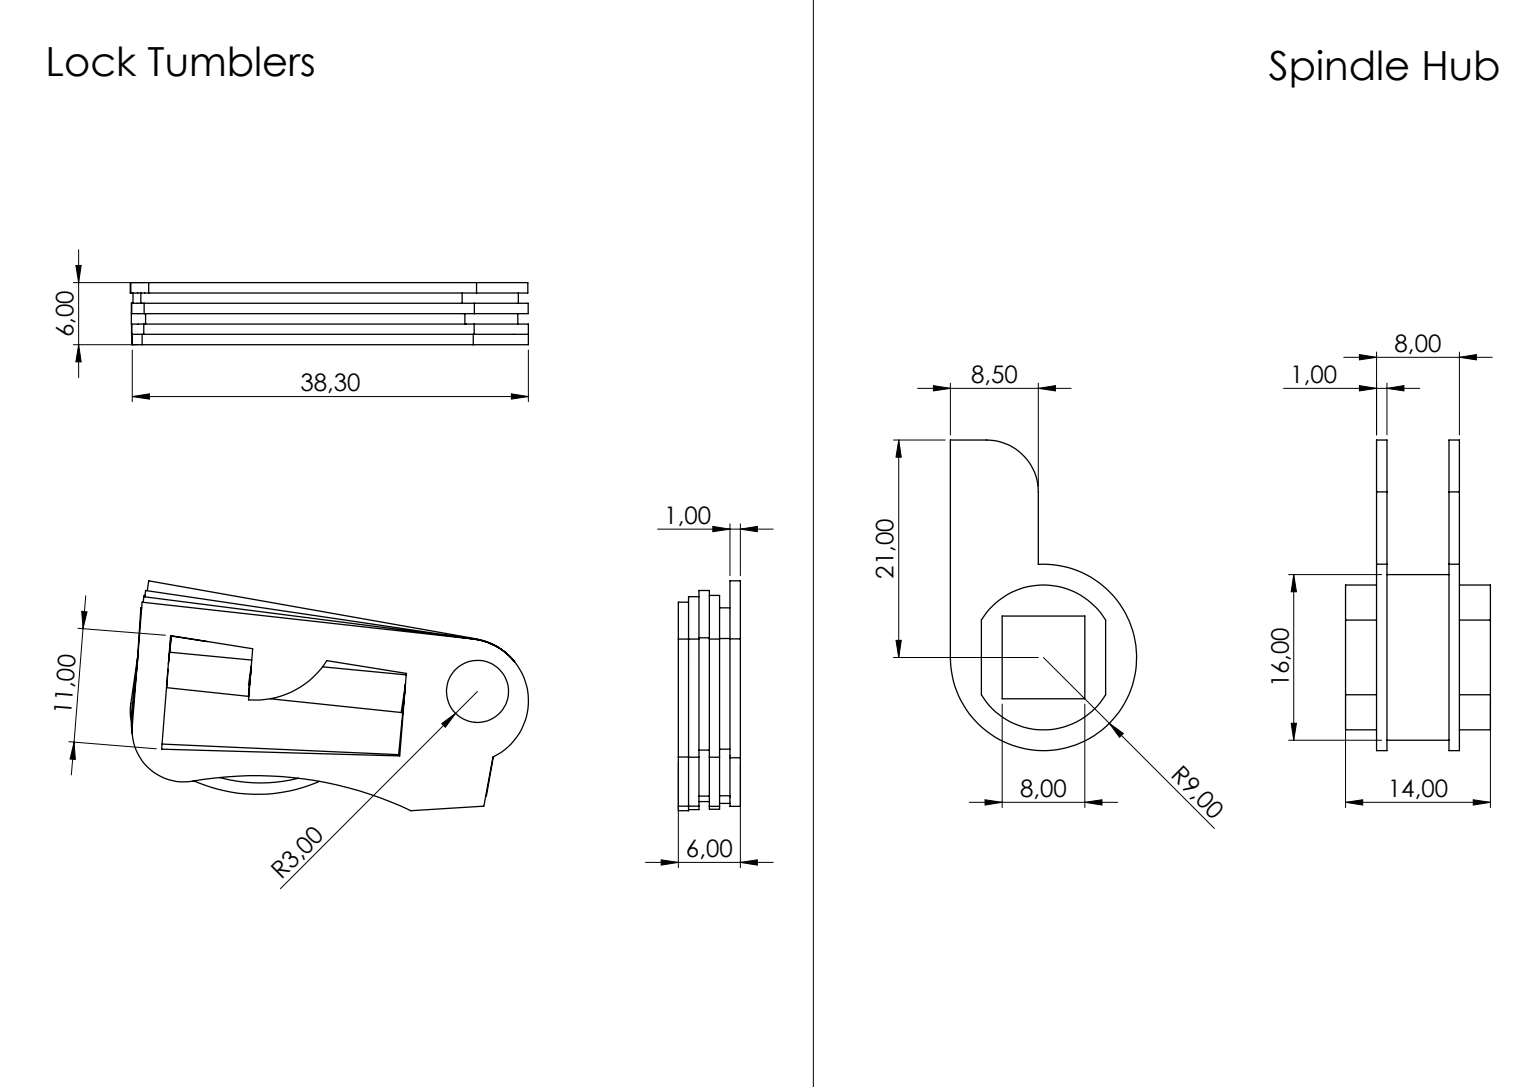
ISO-10303-21;
HEADER;
FILE_DESCRIPTION (('STEP AP214'),
    '1' );
FILE_NAME ('Lock Tumblers.step',
    '2026-10-06T13:23:30',
    ( '' ),
    ( '' ),
    'SwSTEP 2.0',
    'SolidWorks 2020',
    '' );
FILE_SCHEMA (( 'AUTOMOTIVE_DESIGN' ));
ENDSEC;

DATA;
#9=LINE ( 'NONE', #19761, #1381 ) ;
#17=VECTOR ( 'NONE', #19861, 1000.000000000000114 ) ;
#19=EDGE_CURVE ( 'NONE', #10851, #14365, #21344, .T. ) ;
#28=LINE ( 'NONE', #12848, #13253 ) ;
#29=DIRECTION ( 'NONE',  ( -2.842170943040000002E-14, -3.552713678800000097E-13, -1.000000000000000000 ) ) ;
#30=VERTEX_POINT ( 'NONE', #23278 ) ;
#34=VERTEX_POINT ( 'NONE', #8858 ) ;
#37=CARTESIAN_POINT ( 'NONE',  ( 5.631397321050000571, -17.85059010000000157, -146.5552959529999839 ) ) ;
#50=EDGE_CURVE ( 'NONE', #22537, #320, #23237, .T. ) ;
#60=AXIS2_PLACEMENT_3D ( 'NONE', #23173, #12444, #1408 ) ;
#64=LINE ( 'NONE', #5521, #16191 ) ;
#66=PLANE ( 'NONE',  #21173 ) ;
#67=CARTESIAN_POINT ( 'NONE',  ( 15.97954986339999905, -26.72957102550000030, -142.5552959529999839 ) ) ;
#69=CARTESIAN_POINT ( 'NONE',  ( -4.946601369560000627, -23.77962690289999870, -143.5552959529999839 ) ) ;
#80=CARTESIAN_POINT ( 'NONE',  ( 1.600095057559999923, -18.40127899619999852, -146.5552959529999839 ) ) ;
#81=VECTOR ( 'NONE', #14435, 1000.000000000000114 ) ;
#82=ORIENTED_EDGE ( 'NONE', *, *, #12596, .T. ) ;
#87=ORIENTED_EDGE ( 'NONE', *, *, #14036, .T. ) ;
#93=DIRECTION ( 'NONE',  ( -0.9892101392001054760, 0.1465035852930155480, 4.471739159800472250E-12 ) ) ;
#97=AXIS2_PLACEMENT_3D ( 'NONE', #8071, #2741, #23074 ) ;
#98=EDGE_CURVE ( 'NONE', #6545, #18690, #5646, .T. ) ;
#101=ORIENTED_EDGE ( 'NONE', *, *, #18336, .T. ) ;
#109=EDGE_CURVE ( 'NONE', #2866, #16847, #2210, .T. ) ;
#115=FACE_OUTER_BOUND ( 'NONE', #19032, .T. ) ;
#117=CARTESIAN_POINT ( 'NONE',  ( -4.959431410700000598, -23.66636161550000139, -146.0552959529999839 ) ) ;
#118=AXIS2_PLACEMENT_3D ( 'NONE', #14379, #10436, #6880 ) ;
#121=ORIENTED_EDGE ( 'NONE', *, *, #3001, .T. ) ;
#122=CARTESIAN_POINT ( 'NONE',  ( -4.160432423080000497, -28.71743394529999804, -144.5552959529999839 ) ) ;
#124=ORIENTED_EDGE ( 'NONE', *, *, #13380, .T. ) ;
#125=LINE ( 'NONE', #11042, #20030 ) ;
#129=DIRECTION ( 'NONE',  ( -0.9896415801065050477, 0.1435602414469278887, 8.992806499463764746E-12 ) ) ;
#133=CARTESIAN_POINT ( 'NONE',  ( 5.631397321050000571, -17.85059010000000157, -146.5552959529999839 ) ) ;
#152=PLANE ( 'NONE',  #286 ) ;
#164=CARTESIAN_POINT ( 'NONE',  ( -9.056357402059999728, -12.43025388040000045, -147.5552959529999839 ) ) ;
#173=DIRECTION ( 'NONE',  ( -0.09606172499277214338, -0.9953753789357123738, 8.234154099303244678E-13 ) ) ;
#177=EDGE_CURVE ( 'NONE', #22553, #21627, #7661, .T. ) ;
#189=ORIENTED_EDGE ( 'NONE', *, *, #7703, .T. ) ;
#207=ORIENTED_EDGE ( 'NONE', *, *, #948, .T. ) ;
#215=ORIENTED_EDGE ( 'NONE', *, *, #20592, .F. ) ;
#218=LINE ( 'NONE', #15834, #14813 ) ;
#222=ADVANCED_FACE ( 'NONE', ( #11458 ), #4098, .F. ) ;
#224=ORIENTED_EDGE ( 'NONE', *, *, #1037, .F. ) ;
#233=CARTESIAN_POINT ( 'NONE',  ( -6.601136089949999786, -20.10368962670000315, -144.5552959529999839 ) ) ;
#243=CARTESIAN_POINT ( 'NONE',  ( -9.347107914279998653, -17.32706600430000066, -144.5552959529999839 ) ) ;
#245=VECTOR ( 'NONE', #2038, 1000.000000000000114 ) ;
#249=LINE ( 'NONE', #5710, #16739 ) ;
#257=LINE ( 'NONE', #7499, #9038 ) ;
#259=VECTOR ( 'NONE', #18453, 1000.000000000000114 ) ;
#263=CARTESIAN_POINT ( 'NONE',  ( -9.923478264230000789, -23.29931827799999766, -144.5552959529999839 ) ) ;
#265=PLANE ( 'NONE',  #18891 ) ;
#272=VECTOR ( 'NONE', #12599, 1000.000000000000227 ) ;
#275=FACE_OUTER_BOUND ( 'NONE', #1405, .T. ) ;
#286=AXIS2_PLACEMENT_3D ( 'NONE', #3950, #12631, #10950 ) ;
#287=CARTESIAN_POINT ( 'NONE',  ( -9.969904307360000217, -22.67446893780000039, -144.5552959529999839 ) ) ;
#302=EDGE_LOOP ( 'NONE', ( #10238, #8735, #12930, #17915, #645, #16858 ) ) ;
#303=EDGE_CURVE ( 'NONE', #11439, #22823, #3876, .T. ) ;
#320=VERTEX_POINT ( 'NONE', #3034 ) ;
#323=FACE_OUTER_BOUND ( 'NONE', #460, .T. ) ;
#324=ORIENTED_EDGE ( 'NONE', *, *, #8627, .T. ) ;
#325=CARTESIAN_POINT ( 'NONE',  ( -9.434278515689999978, -18.41834002140000237, -147.5552959529999839 ) ) ;
#332=ADVANCED_FACE ( 'NONE', ( #22541 ), #3148, .T. ) ;
#342=DIRECTION ( 'NONE',  ( 0.02818224575639410520, 0.9996028016287901163, -8.199401781418279957E-13 ) ) ;
#343=VECTOR ( 'NONE', #12000, 1000.000000000000000 ) ;
#345=ORIENTED_EDGE ( 'NONE', *, *, #18029, .T. ) ;
#353=AXIS2_PLACEMENT_3D ( 'NONE', #12297, #17774, #23258 ) ;
#356=CARTESIAN_POINT ( 'NONE',  ( -8.296392858609999976, -9.821782169089999570, -148.5552959529999839 ) ) ;
#361=VERTEX_POINT ( 'NONE', #4450 ) ;
#369=DIRECTION ( 'NONE',  ( -2.839308199620000013E-14, -3.568879590630000244E-13, -1.000000000000000000 ) ) ;
#370=ORIENTED_EDGE ( 'NONE', *, *, #23215, .F. ) ;
#377=EDGE_CURVE ( 'NONE', #16716, #11246, #12757, .T. ) ;
#400=CIRCLE ( 'NONE', #3432, 2.999999999999999112 ) ;
#401=ORIENTED_EDGE ( 'NONE', *, *, #15313, .F. ) ;
#404=VERTEX_POINT ( 'NONE', #21825 ) ;
#405=CYLINDRICAL_SURFACE ( 'NONE', #14494, 8.176568160360000448 ) ;
#410=CARTESIAN_POINT ( 'NONE',  ( -7.129475577410000042, -25.57825421080000083, -144.0552959529999839 ) ) ;
#428=AXIS2_PLACEMENT_3D ( 'NONE', #17687, #19484, #10762 ) ;
#440=ADVANCED_FACE ( 'NONE', ( #21467 ), #14562, .T. ) ;
#449=ORIENTED_EDGE ( 'NONE', *, *, #3663, .T. ) ;
#451=ORIENTED_EDGE ( 'NONE', *, *, #12079, .F. ) ;
#456=LINE ( 'NONE', #20555, #2007 ) ;
#460=EDGE_LOOP ( 'NONE', ( #22587, #8189, #13653, #11072, #16704 ) ) ;
#463=VECTOR ( 'NONE', #13106, 999.9999999999998863 ) ;
#470=EDGE_CURVE ( 'NONE', #2284, #2388, #4261, .T. ) ;
#473=VERTEX_POINT ( 'NONE', #1610 ) ;
#475=ADVANCED_FACE ( 'NONE', ( #8830 ), #16110, .F. ) ;
#478=FACE_OUTER_BOUND ( 'NONE', #722, .T. ) ;
#490=LINE ( 'NONE', #2397, #14405 ) ;
#494=DIRECTION ( 'NONE',  ( 8.955190032050000935E-12, -9.104778821549999739E-13, 1.000000000000000000 ) ) ;
#496=ORIENTED_EDGE ( 'NONE', *, *, #9897, .T. ) ;
#497=EDGE_CURVE ( 'NONE', #7372, #10073, #14436, .T. ) ;
#498=MECHANICAL_DESIGN_GEOMETRIC_PRESENTATION_REPRESENTATION('',(#20638),#15318);
#512=ADVANCED_FACE ( 'NONE', ( #5969 ), #11083, .F. ) ;
#513=EDGE_CURVE ( 'NONE', #11545, #10772, #7749, .T. ) ;
#516=PRODUCT_DEFINITION_FORMATION_WITH_SPECIFIED_SOURCE ( 'ANY', '', #19655, .NOT_KNOWN. ) ;
#518=ORIENTED_EDGE ( 'NONE', *, *, #18360, .T. ) ;
#530=CARTESIAN_POINT ( 'NONE',  ( -6.547730170579999509, -18.66441632429999942, -147.5552959529999839 ) ) ;
#552=VECTOR ( 'NONE', #14058, 1000.000000000000000 ) ;
#558=DIRECTION ( 'NONE',  ( 0.05349466063429310358, 0.9985681355238719137, -1.093104632299860501E-13 ) ) ;
#561=ORIENTED_EDGE ( 'NONE', *, *, #19, .F. ) ;
#569=CARTESIAN_POINT ( 'NONE',  ( 4.352290413739999586, -26.01556969399999986, -145.5552959529999839 ) ) ;
#574=EDGE_CURVE ( 'NONE', #10851, #1178, #9171, .T. ) ;
#578=CARTESIAN_POINT ( 'NONE',  ( -6.264930628975839966, -16.71491984542973341, -147.5552959529461816 ) ) ;
#579=VECTOR ( 'NONE', #12352, 1000.000000000000114 ) ;
#580=DIRECTION ( 'NONE',  ( 1.000000000000000000, 0.000000000000000000, -1.522591576628786004E-13 ) ) ;
#588=ORIENTED_EDGE ( 'NONE', *, *, #13323, .F. ) ;
#589=LINE ( 'NONE', #22831, #9470 ) ;
#593=LINE ( 'NONE', #4279, #23134 ) ;
#599=DIRECTION ( 'NONE',  ( 4.430318231640945063E-12, -6.100259101492280662E-13, 1.000000000000000000 ) ) ;
#619=DIRECTION ( 'NONE',  ( -1.525446435830000185E-13, -8.171241461240000022E-13, -1.000000000000000000 ) ) ;
#621=DIRECTION ( 'NONE',  ( 1.000000000000000000, 0.000000000000000000, -4.510774274160000731E-12 ) ) ;
#622=FACE_OUTER_BOUND ( 'NONE', #19220, .T. ) ;
#627=DIRECTION ( 'NONE',  ( 0.9990052710704846461, -0.04459224566432164194, -1.160036675700561719E-13 ) ) ;
#632=VECTOR ( 'NONE', #2081, 1000.000000000000114 ) ;
#642=DIRECTION ( 'NONE',  ( 0.9990052710704846461, -0.04459224566432164194, -1.160036675700561719E-13 ) ) ;
#645=ORIENTED_EDGE ( 'NONE', *, *, #21775, .T. ) ;
#655=DIRECTION ( 'NONE',  ( 2.839308199620000013E-14, 3.568879590630000244E-13, 1.000000000000000000 ) ) ;
#667=ORIENTED_EDGE ( 'NONE', *, *, #18339, .F. ) ;
#672=LINE ( 'NONE', #8257, #20839 ) ;
#674=EDGE_LOOP ( 'NONE', ( #13508, #15033, #13775, #6801 ) ) ;
#685=ORIENTED_EDGE ( 'NONE', *, *, #13914, .T. ) ;
#689=LINE ( 'NONE', #22455, #8666 ) ;
#694=AXIS2_PLACEMENT_3D ( 'NONE', #20611, #4769, #621 ) ;
#698=ORIENTED_EDGE ( 'NONE', *, *, #6854, .T. ) ;
#701=CARTESIAN_POINT ( 'NONE',  ( -9.282104535849999394, -16.71402168319999859, -144.5552959529999839 ) ) ;
#703=DIRECTION ( 'NONE',  ( 0.1000233216789610108, 0.9949850929136109245, -3.588240815588595806E-13 ) ) ;
#712=VERTEX_POINT ( 'NONE', #6671 ) ;
#720=CARTESIAN_POINT ( 'NONE',  ( 24.89581725840000104, -26.85672394480000236, -144.5552959529999839 ) ) ;
#722=EDGE_LOOP ( 'NONE', ( #8412, #1698, #20815, #12753, #12822 ) ) ;
#727=ORIENTED_EDGE ( 'NONE', *, *, #8627, .F. ) ;
#732=DIRECTION ( 'NONE',  ( 1.527666881879999979E-13, 8.171241461240000022E-13, 1.000000000000000000 ) ) ;
#735=CARTESIAN_POINT ( 'NONE',  ( 25.00000852249999994, -26.83294714660000224, -143.5552959529999839 ) ) ;
#737=EDGE_CURVE ( 'NONE', #2750, #10162, #17272, .T. ) ;
#744=EDGE_CURVE ( 'NONE', #22823, #11439, #6921, .T. ) ;
#747=DIRECTION ( 'NONE',  ( 0.9944529286486341046, -0.1051825684329612265, -4.469111776238355154E-12 ) ) ;
#749=CARTESIAN_POINT ( 'NONE',  ( 23.40529971389999986, -31.60139774330000151, -148.5552959529999839 ) ) ;
#753=AXIS2_PLACEMENT_3D ( 'NONE', #701, #11861, #18779 ) ;
#757=CIRCLE ( 'NONE', #2659, 9.999999999999998224 ) ;
#760=VERTEX_POINT ( 'NONE', #3003 ) ;
#773=DIRECTION ( 'NONE',  ( 1.000000000000000000, 0.000000000000000000, -4.429789868254375404E-12 ) ) ;
#776=AXIS2_PLACEMENT_3D ( 'NONE', #3674, #5214, #14152 ) ;
#792=EDGE_CURVE ( 'NONE', #34, #13141, #18820, .T. ) ;
#799=ADVANCED_FACE ( 'NONE', ( #15723 ), #13459, .T. ) ;
#803=DIRECTION ( 'NONE',  ( 8.955190032048950803E-12, -9.104778821523669707E-13, 1.000000000000000000 ) ) ;
#807=VECTOR ( 'NONE', #9050, 1000.000000000000227 ) ;
#808=ORIENTED_EDGE ( 'NONE', *, *, #13766, .F. ) ;
#811=DIRECTION ( 'NONE',  ( 1.000000000000000000, 0.000000000000000000, -8.953948693601887499E-12 ) ) ;
#817=DIRECTION ( 'NONE',  ( -0.9968185442904001770, 0.07970438983373183406, 8.881784197001251061E-14 ) ) ;
#819=EDGE_CURVE ( 'NONE', #5226, #404, #5017, .T. ) ;
#821=ADVANCED_FACE ( 'NONE', ( #16081 ), #23100, .T. ) ;
#832=DIRECTION ( 'NONE',  ( -0.1739442350240419932, -0.9847555042252370550, 8.300754441162000146E-13 ) ) ;
#833=EDGE_LOOP ( 'NONE', ( #16768, #6878, #10888, #18161, #3058, #10823 ) ) ;
#834=PLANE ( 'NONE',  #6066 ) ;
#836=ORIENTED_EDGE ( 'NONE', *, *, #936, .F. ) ;
#842=CARTESIAN_POINT ( 'NONE',  ( -9.157754307299999397, -15.75963164970000108, -148.5552959529999839 ) ) ;
#846=DIRECTION ( 'NONE',  ( -0.07970438983373200059, -0.9968185442904001770, 8.268372250843320857E-13 ) ) ;
#852=DIRECTION ( 'NONE',  ( 1.526468026909860048E-13, 8.159623473498529972E-13, 1.000000000000000000 ) ) ;
#854=EDGE_CURVE ( 'NONE', #14669, #14970, #11031, .T. ) ;
#859=DIRECTION ( 'NONE',  ( 0.000000000000000000, -1.000000000000000000, 8.159623473500000156E-13 ) ) ;
#865=VECTOR ( 'NONE', #15700, 1000.000000000000000 ) ;
#866=DIRECTION ( 'NONE',  ( 0.000000000000000000, 1.093106450072369968E-12, -1.000000000000000000 ) ) ;
#874=ORIENTED_EDGE ( 'NONE', *, *, #177, .T. ) ;
#888=DIRECTION ( 'NONE',  ( -0.9892101392001054760, 0.1465035852930155480, 4.471739159800472250E-12 ) ) ;
#890=LINE ( 'NONE', #6109, #6665 ) ;
#900=ORIENTED_EDGE ( 'NONE', *, *, #13310, .T. ) ;
#914=CARTESIAN_POINT ( 'NONE',  ( 24.11847952820000174, -31.58456057200000089, -143.0552959529999839 ) ) ;
#917=ORIENTED_EDGE ( 'NONE', *, *, #16657, .T. ) ;
#919=VERTEX_POINT ( 'NONE', #10579 ) ;
#922=ORIENTED_EDGE ( 'NONE', *, *, #6201, .F. ) ;
#923=AXIS2_PLACEMENT_3D ( 'NONE', #3964, #20620, #5970 ) ;
#929=DIRECTION ( 'NONE',  ( 0.9957290851625899553, -0.09232328504376198508, -9.001390970786290700E-12 ) ) ;
#930=ORIENTED_EDGE ( 'NONE', *, *, #18567, .F. ) ;
#936=EDGE_CURVE ( 'NONE', #19018, #10871, #218, .T. ) ;
#948=EDGE_CURVE ( 'NONE', #8156, #9207, #7576, .T. ) ;
#955=CARTESIAN_POINT ( 'NONE',  ( 2.218297500559999857, -15.44723318490000175, -146.5552959529999839 ) ) ;
#956=EDGE_CURVE ( 'NONE', #22736, #2628, #6149, .T. ) ;
#959=EDGE_CURVE ( 'NONE', #19705, #16855, #22573, .T. ) ;
#960=CARTESIAN_POINT ( 'NONE',  ( 1.829659965300000080, -16.02499107890000118, -143.5552959529999839 ) ) ;
#961=AXIS2_PLACEMENT_3D ( 'NONE', #19818, #21604, #5064 ) ;
#962=ORIENTED_EDGE ( 'NONE', *, *, #13286, .T. ) ;
#966=LINE ( 'NONE', #6082, #22322 ) ;
#975=VECTOR ( 'NONE', #19311, 1000.000000000000114 ) ;
#976=ORIENTED_EDGE ( 'NONE', *, *, #17520, .F. ) ;
#987=DIRECTION ( 'NONE',  ( 0.000000000000000000, 1.093106450072369968E-12, -1.000000000000000000 ) ) ;
#998=CARTESIAN_POINT ( 'NONE',  ( 24.75935218339999722, -28.32938697159999819, -147.5552959529999839 ) ) ;
#1019=CARTESIAN_POINT ( 'NONE',  ( 5.276897646250000129, -21.39828525539999760, -145.5552959529999839 ) ) ;
#1023=LINE ( 'NONE', #8251, #17696 ) ;
#1037=EDGE_CURVE ( 'NONE', #9207, #2750, #18595, .T. ) ;
#1038=VERTEX_POINT ( 'NONE', #11600 ) ;
#1040=ORIENTED_EDGE ( 'NONE', *, *, #20103, .F. ) ;
#1045=LINE ( 'NONE', #22814, #19399 ) ;
#1049=DIRECTION ( 'NONE',  ( 1.526468026909999897E-13, 8.159623473500000156E-13, 1.000000000000000000 ) ) ;
#1051=ORIENTED_EDGE ( 'NONE', *, *, #16098, .F. ) ;
#1052=CIRCLE ( 'NONE', #17006, 15.00000000000000000 ) ;
#1058=DIRECTION ( 'NONE',  ( 0.09232328504376198508, 0.9957290851625899553, 7.981674670826710110E-14 ) ) ;
#1065=EDGE_CURVE ( 'NONE', #12475, #2580, #7691, .T. ) ;
#1066=EDGE_LOOP ( 'NONE', ( #14610, #17073, #1898, #21878, #8834 ) ) ;
#1068=PLANE ( 'NONE',  #6979 ) ;
#1076=ORIENTED_EDGE ( 'NONE', *, *, #1211, .T. ) ;
#1082=ORIENTED_EDGE ( 'NONE', *, *, #12807, .T. ) ;
#1090=CARTESIAN_POINT ( 'NONE',  ( -8.734077015120000453, -11.22642389220000148, -146.5552959529999839 ) ) ;
#1093=CARTESIAN_POINT ( 'NONE',  ( -5.758148842640000709, -13.22138763369999914, -148.5552959529999839 ) ) ;
#1095=CARTESIAN_POINT ( 'NONE',  ( 1.354168148130000082, -20.95195702430000040, -143.5552959529999839 ) ) ;
#1101=DIRECTION ( 'NONE',  ( 1.526468026909999897E-13, 8.159623473500000156E-13, 1.000000000000000000 ) ) ;
#1106=DIRECTION ( 'NONE',  ( -0.06298685227120542907, -0.9980143568310855251, 1.515824502950130739E-13 ) ) ;
#1135=ORIENTED_EDGE ( 'NONE', *, *, #2562, .F. ) ;
#1137=DIRECTION ( 'NONE',  ( 4.518783361002970486E-12, 0.000000000000000000, 1.000000000000000000 ) ) ;
#1140=VERTEX_POINT ( 'NONE', #21622 ) ;
#1143=CARTESIAN_POINT ( 'NONE',  ( 7.558347240399999833, -12.62842008530000015, -148.5552959529999839 ) ) ;
#1144=ORIENTED_EDGE ( 'NONE', *, *, #8369, .T. ) ;
#1153=CARTESIAN_POINT ( 'NONE',  ( -9.434278515689999978, -18.41834002140000237, -146.5552959529999839 ) ) ;
#1157=AXIS2_PLACEMENT_3D ( 'NONE', #117, #1784, #12704 ) ;
#1161=DIRECTION ( 'NONE',  ( 1.000000000000000000, 0.000000000000000000, 0.000000000000000000 ) ) ;
#1166=DIRECTION ( 'NONE',  ( 0.9990052710704846461, -0.04459224566432164194, -1.160036675700561719E-13 ) ) ;
#1168=VERTEX_POINT ( 'NONE', #23513 ) ;
#1169=CARTESIAN_POINT ( 'NONE',  ( 21.79964646190000011, -30.87346604779999737, -144.5552959529999839 ) ) ;
#1175=VECTOR ( 'NONE', #18133, 999.9999999999998863 ) ;
#1178=VERTEX_POINT ( 'NONE', #7211 ) ;
#1185=DIRECTION ( 'NONE',  ( 0.4472766253858966867, 0.8943956732807937238, -3.322738909413859124E-13 ) ) ;
#1193=LINE ( 'NONE', #15225, #13000 ) ;
#1200=CARTESIAN_POINT ( 'NONE',  ( 2.068499633510000102, -14.99362786250000035, -147.5552959529999839 ) ) ;
#1203=LINE ( 'NONE', #15346, #6548 ) ;
#1204=ORIENTED_EDGE ( 'NONE', *, *, #16657, .F. ) ;
#1206=LINE ( 'NONE', #15458, #23527 ) ;
#1208=VECTOR ( 'NONE', #21514, 1000.000000000000114 ) ;
#1211=EDGE_CURVE ( 'NONE', #6134, #15113, #9565, .T. ) ;
#1221=CARTESIAN_POINT ( 'NONE',  ( 12.81474735470000148, -17.96536370379999781, -144.5552959529999839 ) ) ;
#1224=ORIENTED_EDGE ( 'NONE', *, *, #1675, .T. ) ;
#1228=CARTESIAN_POINT ( 'NONE',  ( -6.120427241202767377, -15.12266568073683537, -143.5552959530020019 ) ) ;
#1250=CARTESIAN_POINT ( 'NONE',  ( 22.33963087269999903, -30.94765732060000119, -146.5552959529999839 ) ) ;
#1251=CARTESIAN_POINT ( 'NONE',  ( -9.157754307290000284, -15.75963164970000108, -147.5552959529999839 ) ) ;
#1252=EDGE_CURVE ( 'NONE', #14970, #1892, #16838, .T. ) ;
#1258=AXIS2_PLACEMENT_3D ( 'NONE', #6292, #9969, #17243 ) ;
#1279=ORIENTED_EDGE ( 'NONE', *, *, #2845, .T. ) ;
#1283=CARTESIAN_POINT ( 'NONE',  ( 2.016283561950000358, -13.16498300129999954, -143.5552959529999839 ) ) ;
#1303=CARTESIAN_POINT ( 'NONE',  ( -7.337311498540000088, -24.10744501490000147, -147.5552959529999839 ) ) ;
#1304=ORIENTED_EDGE ( 'NONE', *, *, #5149, .F. ) ;
#1309=CARTESIAN_POINT ( 'NONE',  ( -9.812199629320000227, -24.40642616239999896, -147.5552959529999839 ) ) ;
#1324=FACE_OUTER_BOUND ( 'NONE', #21450, .T. ) ;
#1338=DIRECTION ( 'NONE',  ( 2.839308199620000013E-14, 3.568879590630000244E-13, 1.000000000000000000 ) ) ;
#1378=DIRECTION ( 'NONE',  ( -0.9840552701943220404, 0.1778629393740580045, -3.651917849741195385E-14 ) ) ;
#1380=VERTEX_POINT ( 'NONE', #20883 ) ;
#1381=VECTOR ( 'NONE', #3456, 1000.000000000000000 ) ;
#1383=VECTOR ( 'NONE', #7873, 1000.000000000000114 ) ;
#1385=ADVANCED_FACE ( 'NONE', ( #15865 ), #13608, .F. ) ;
#1388=LINE ( 'NONE', #17678, #17059 ) ;
#1389=LINE ( 'NONE', #3062, #2353 ) ;
#1401=EDGE_CURVE ( 'NONE', #21066, #12006, #19779, .T. ) ;
#1405=EDGE_LOOP ( 'NONE', ( #12527, #20995, #14025, #12342, #16570, #13119 ) ) ;
#1408=DIRECTION ( 'NONE',  ( 0.000000000000000000, -1.000000000000000000, 3.568879590630000244E-13 ) ) ;
#1412=EDGE_CURVE ( 'NONE', #2388, #15779, #6827, .T. ) ;
#1414=ORIENTED_EDGE ( 'NONE', *, *, #13034, .F. ) ;
#1425=DIRECTION ( 'NONE',  ( 0.09606172499277226828, 0.9953753789357124848, -8.277822871607614780E-13 ) ) ;
#1427=VERTEX_POINT ( 'NONE', #8372 ) ;
#1428=LINE ( 'NONE', #7357, #3054 ) ;
#1430=ORIENTED_EDGE ( 'NONE', *, *, #14481, .F. ) ;
#1436=AXIS2_PLACEMENT_3D ( 'NONE', #3180, #6733, #14352 ) ;
#1458=CARTESIAN_POINT ( 'NONE',  ( -6.165211177139999776, -15.11551140080000089, -142.5552959529999839 ) ) ;
#1460=ORIENTED_EDGE ( 'NONE', *, *, #13738, .F. ) ;
#1462=EDGE_CURVE ( 'NONE', #21680, #8156, #18971, .T. ) ;
#1464=EDGE_LOOP ( 'NONE', ( #4342, #10992, #21636 ) ) ;
#1470=LINE ( 'NONE', #7039, #16255 ) ;
#1484=EDGE_CURVE ( 'NONE', #21680, #6936, #13736, .T. ) ;
#1486=VERTEX_POINT ( 'NONE', #19677 ) ;
#1489=AXIS2_PLACEMENT_3D ( 'NONE', #19639, #18090, #1802 ) ;
#1490=EDGE_CURVE ( 'NONE', #4619, #22505, #18016, .T. ) ;
#1492=FACE_OUTER_BOUND ( 'NONE', #7110, .T. ) ;
#1497=DIRECTION ( 'NONE',  ( 1.526468026909999897E-13, 8.159623473500000156E-13, 1.000000000000000000 ) ) ;
#1499=CARTESIAN_POINT ( 'NONE',  ( 19.75551406279999966, -31.14090339520000228, -145.0552959529999839 ) ) ;
#1503=EDGE_CURVE ( 'NONE', #8311, #21143, #14320, .T. ) ;
#1512=VECTOR ( 'NONE', #929, 1000.000000000000114 ) ;
#1515=CARTESIAN_POINT ( 'NONE',  ( -9.282104535849999394, -16.71402168319999859, -144.5552959529999839 ) ) ;
#1524=AXIS2_PLACEMENT_3D ( 'NONE', #17663, #8596, #15869 ) ;
#1526=EDGE_LOOP ( 'NONE', ( #20689, #14688, #9788, #17546 ) ) ;
#1532=DIRECTION ( 'NONE',  ( 1.000000000000000000, 0.000000000000000000, -2.775557561562891351E-14 ) ) ;
#1535=FACE_OUTER_BOUND ( 'NONE', #6075, .T. ) ;
#1543=EDGE_CURVE ( 'NONE', #11590, #6997, #9059, .T. ) ;
#1544=DIRECTION ( 'NONE',  ( 4.430318231639999944E-12, -6.100259101500000139E-13, 1.000000000000000000 ) ) ;
#1548=CIRCLE ( 'NONE', #8343, 6.000000000000001776 ) ;
#1549=ORIENTED_EDGE ( 'NONE', *, *, #22549, .F. ) ;
#1550=CIRCLE ( 'NONE', #22056, 35.00000000000000000 ) ;
#1554=DIRECTION ( 'NONE',  ( 2.842170943040000002E-14, 3.552713678800000097E-13, 1.000000000000000000 ) ) ;
#1556=DIRECTION ( 'NONE',  ( 1.000000000000000000, 0.000000000000000000, -4.510774274160000731E-12 ) ) ;
#1563=AXIS2_PLACEMENT_3D ( 'NONE', #3226, #10458, #5121 ) ;
#1571=CARTESIAN_POINT ( 'NONE',  ( -6.599319970649999867, -19.98386714700000155, -146.5552959529999839 ) ) ;
#1574=DIRECTION ( 'NONE',  ( -0.9840552701943220404, 0.1778629393740580045, -3.651917849741195385E-14 ) ) ;
#1590=VERTEX_POINT ( 'NONE', #19566 ) ;
#1596=LINE ( 'NONE', #17523, #16597 ) ;
#1598=ORIENTED_EDGE ( 'NONE', *, *, #2438, .F. ) ;
#1609=FACE_OUTER_BOUND ( 'NONE', #5677, .T. ) ;
#1610=CARTESIAN_POINT ( 'NONE',  ( -9.310255235759342440, -16.95797460217655939, -145.5552959530000692 ) ) ;
#1611=DIRECTION ( 'NONE',  ( 1.000000000000000000, 0.000000000000000000, -4.429789868254373788E-12 ) ) ;
#1619=CIRCLE ( 'NONE', #13756, 6.000000000000001776 ) ;
#1640=DIRECTION ( 'NONE',  ( -0.06298685227120542907, -0.9980143568310855251, 1.534772309240130738E-13 ) ) ;
#1642=CARTESIAN_POINT ( 'NONE',  ( -9.282104535849999394, -16.71402168319999859, -144.5552959529999839 ) ) ;
#1649=AXIS2_PLACEMENT_3D ( 'NONE', #5854, #4424, #17156 ) ;
#1652=EDGE_LOOP ( 'NONE', ( #22705, #449, #5626, #4466, #23537, #11215 ) ) ;
#1654=ORIENTED_EDGE ( 'NONE', *, *, #574, .F. ) ;
#1657=VERTEX_POINT ( 'NONE', #8323 ) ;
#1658=CARTESIAN_POINT ( 'NONE',  ( -6.599319970649999867, -19.98386714700000155, -146.5552959529999839 ) ) ;
#1670=CARTESIAN_POINT ( 'NONE',  ( 24.55924402540000173, -29.20875385929999979, -142.5552959529999839 ) ) ;
#1672=DIRECTION ( 'NONE',  ( 1.337196879809910072E-12, 0.000000000000000000, -1.000000000000000000 ) ) ;
#1674=CARTESIAN_POINT ( 'NONE',  ( 5.347956485829999274, -22.34165470570000167, -146.5552959529999839 ) ) ;
#1675=EDGE_CURVE ( 'NONE', #7250, #3831, #15948, .T. ) ;
#1681=DIRECTION ( 'NONE',  ( -0.1000233216789610108, -0.9949850929136109245, 3.591470555298595137E-13 ) ) ;
#1682=ORIENTED_EDGE ( 'NONE', *, *, #2724, .F. ) ;
#1686=CARTESIAN_POINT ( 'NONE',  ( -9.282104535860000283, -16.71402168319999859, -145.5552959529999839 ) ) ;
#1689=EDGE_CURVE ( 'NONE', #2706, #23117, #19526, .T. ) ;
#1691=CARTESIAN_POINT ( 'NONE',  ( -6.083910486889999802, -15.16899799649999991, -145.0552959529999839 ) ) ;
#1698=ORIENTED_EDGE ( 'NONE', *, *, #12513, .T. ) ;
#1708=CARTESIAN_POINT ( 'NONE',  ( 1.352544480119999948, -20.86379603889999856, -146.0552959529999839 ) ) ;
#1717=VERTEX_POINT ( 'NONE', #19163 ) ;
#1726=ORIENTED_EDGE ( 'NONE', *, *, #22913, .F. ) ;
#1730=DIRECTION ( 'NONE',  ( 1.000000000000000000, 0.000000000000000000, -8.955190032050000935E-12 ) ) ;
#1732=LINE ( 'NONE', #16574, #20010 ) ;
#1739=ADVANCED_FACE ( 'NONE', ( #22976 ), #6661, .F. ) ;
#1766=EDGE_CURVE ( 'NONE', #14876, #5894, #19763, .T. ) ;
#1779=VERTEX_POINT ( 'NONE', #7375 ) ;
#1781=LINE ( 'NONE', #7356, #21776 ) ;
#1784=DIRECTION ( 'NONE',  ( 2.839308199624610116E-14, 3.568879590629954805E-13, 1.000000000000000000 ) ) ;
#1785=DIRECTION ( 'NONE',  ( 4.430318231639999944E-12, -6.100259101500000139E-13, 1.000000000000000000 ) ) ;
#1795=EDGE_LOOP ( 'NONE', ( #13048, #3731 ) ) ;
#1800=CARTESIAN_POINT ( 'NONE',  ( -9.434278515689999978, -18.41834002140000237, -146.5552959529999839 ) ) ;
#1802=DIRECTION ( 'NONE',  ( 1.000000000000000000, 0.000000000000000000, -1.527536832333223921E-13 ) ) ;
#1810=DIRECTION ( 'NONE',  ( 0.000000000000000000, -1.000000000000000000, 3.568879590630000244E-13 ) ) ;
#1812=ORIENTED_EDGE ( 'NONE', *, *, #10380, .T. ) ;
#1817=ADVANCED_FACE ( 'NONE', ( #9019 ), #10924, .F. ) ;
#1826=EDGE_CURVE ( 'NONE', #18313, #11439, #12479, .T. ) ;
#1828=AXIS2_PLACEMENT_3D ( 'NONE', #8316, #5953, #13686 ) ;
#1839=DIRECTION ( 'NONE',  ( 0.000000000000000000, -1.000000000000000000, 8.159623473500000156E-13 ) ) ;
#1847=EDGE_CURVE ( 'NONE', #21627, #4947, #18646, .T. ) ;
#1851=ADVANCED_FACE ( 'NONE', ( #17975 ), #16305, .F. ) ;
#1862=CIRCLE ( 'NONE', #9426, 2.999999999999999112 ) ;
#1867=DIRECTION ( 'NONE',  ( 4.500711553433139826E-12, 0.000000000000000000, 1.000000000000000000 ) ) ;
#1874=DIRECTION ( 'NONE',  ( 0.9934078757590584230, -0.1146332952500066366, -4.471042303700262431E-12 ) ) ;
#1875=ADVANCED_BREP_SHAPE_REPRESENTATION ( '', ( #11538, #5025 ), #13402 ) ;
#1876=ORIENTED_EDGE ( 'NONE', *, *, #7732, .F. ) ;
#1884=AXIS2_PLACEMENT_3D ( 'NONE', #9269, #18337, #3821 ) ;
#1889=LINE ( 'NONE', #19608, #13521 ) ;
#1890=ORIENTED_EDGE ( 'NONE', *, *, #12099, .F. ) ;
#1892=VERTEX_POINT ( 'NONE', #14174 ) ;
#1895=ORIENTED_EDGE ( 'NONE', *, *, #21508, .F. ) ;
#1898=ORIENTED_EDGE ( 'NONE', *, *, #12267, .T. ) ;
#1900=AXIS2_PLACEMENT_3D ( 'NONE', #9741, #20831, #859 ) ;
#1902=ORIENTED_EDGE ( 'NONE', *, *, #14694, .F. ) ;
#1909=CIRCLE ( 'NONE', #8712, 8.176568160360000448 ) ;
#1912=LINE ( 'NONE', #11380, #10974 ) ;
#1913=ORIENTED_EDGE ( 'NONE', *, *, #11237, .T. ) ;
#1920=LINE ( 'NONE', #5476, #245 ) ;
#1922=CIRCLE ( 'NONE', #6467, 5.999999999999998224 ) ;
#1941=ORIENTED_EDGE ( 'NONE', *, *, #3278, .T. ) ;
#1953=CARTESIAN_POINT ( 'NONE',  ( 2.218297500549999857, -15.44723318490000175, -147.5552959529999839 ) ) ;
#1956=LINE ( 'NONE', #5619, #807 ) ;
#1958=PLANE ( 'NONE',  #5768 ) ;
#1966=DIRECTION ( 'NONE',  ( 0.9980143568310856361, -0.06298685227120542907, -4.509810669690387962E-12 ) ) ;
#1977=LINE ( 'NONE', #14924, #8160 ) ;
#1979=ORIENTED_EDGE ( 'NONE', *, *, #20130, .T. ) ;
#1986=DIRECTION ( 'NONE',  ( 0.5768293036180225375, -0.8168647100270319816, -3.053113317719179274E-12 ) ) ;
#1987=ORIENTED_EDGE ( 'NONE', *, *, #13409, .T. ) ;
#1992=ADVANCED_FACE ( 'NONE', ( #15956 ), #10575, .T. ) ;
#1998=VERTEX_POINT ( 'NONE', #16077 ) ;
#2004=AXIS2_PLACEMENT_3D ( 'NONE', #20460, #3814, #4155 ) ;
#2006=VECTOR ( 'NONE', #18307, 1000.000000000000227 ) ;
#2007=VECTOR ( 'NONE', #9698, 1000.000000000000000 ) ;
#2031=VERTEX_POINT ( 'NONE', #14406 ) ;
#2032=DIRECTION ( 'NONE',  ( -0.1146332952500066227, -0.9934078757590583120, -9.710750722050572275E-14 ) ) ;
#2038=DIRECTION ( 'NONE',  ( -0.07970438983373200059, -0.9968185442904001770, 8.268133652483321323E-13 ) ) ;
#2043=DIRECTION ( 'NONE',  ( 0.9980719161006958995, 0.06206811009758109871, -2.049912714059374948E-13 ) ) ;
#2044=EDGE_CURVE ( 'NONE', #6018, #11453, #249, .T. ) ;
#2047=CARTESIAN_POINT ( 'NONE',  ( 20.31210873290000052, -31.32069079449999904, -146.5552959529999839 ) ) ;
#2048=FACE_OUTER_BOUND ( 'NONE', #2108, .T. ) ;
#2050=DIRECTION ( 'NONE',  ( 0.9944529286486341046, -0.1051825684329612265, -4.470295960598355531E-12 ) ) ;
#2051=ORIENTED_EDGE ( 'NONE', *, *, #18360, .F. ) ;
#2054=ORIENTED_EDGE ( 'NONE', *, *, #12849, .F. ) ;
#2063=CARTESIAN_POINT ( 'NONE',  ( 19.75551406279999966, -31.14090339520000228, -144.5552959529999839 ) ) ;
#2073=DIRECTION ( 'NONE',  ( -0.9792968044389154247, 0.2024296638729825848, -4.443945512649620152E-14 ) ) ;
#2078=ORIENTED_EDGE ( 'NONE', *, *, #13262, .T. ) ;
#2081=DIRECTION ( 'NONE',  ( 0.9980719161006958995, 0.06206811009758109871, -2.049912714059374948E-13 ) ) ;
#2085=CIRCLE ( 'NONE', #5489, 5.000000000000000000 ) ;
#2090=ORIENTED_EDGE ( 'NONE', *, *, #20324, .F. ) ;
#2091=ADVANCED_FACE ( 'NONE', ( #22365 ), #7832, .F. ) ;
#2099=EDGE_CURVE ( 'NONE', #14032, #4598, #22248, .T. ) ;
#2108=EDGE_LOOP ( 'NONE', ( #2629, #18054, #13739, #17573 ) ) ;
#2112=VECTOR ( 'NONE', #4682, 1000.000000000000000 ) ;
#2114=VERTEX_POINT ( 'NONE', #2047 ) ;
#2125=DIRECTION ( 'NONE',  ( 0.2229045288590935092, 0.9748402797454081004, -3.928002761761645078E-13 ) ) ;
#2127=EDGE_CURVE ( 'NONE', #2852, #8980, #18335, .T. ) ;
#2128=FACE_OUTER_BOUND ( 'NONE', #4122, .T. ) ;
#2136=EDGE_CURVE ( 'NONE', #4706, #15489, #14753, .T. ) ;
#2150=LINE ( 'NONE', #13074, #11375 ) ;
#2153=VECTOR ( 'NONE', #16879, 1000.000000000000114 ) ;
#2161=ORIENTED_EDGE ( 'NONE', *, *, #17520, .T. ) ;
#2173=ORIENTED_EDGE ( 'NONE', *, *, #18480, .F. ) ;
#2181=AXIS2_PLACEMENT_3D ( 'NONE', #3165, #15655, #10503 ) ;
#2185=ORIENTED_EDGE ( 'NONE', *, *, #5828, .F. ) ;
#2188=FACE_OUTER_BOUND ( 'NONE', #13050, .T. ) ;
#2193=ORIENTED_EDGE ( 'NONE', *, *, #5142, .F. ) ;
#2208=ORIENTED_EDGE ( 'NONE', *, *, #21074, .T. ) ;
#2210=LINE ( 'NONE', #15041, #12594 ) ;
#2213=VERTEX_POINT ( 'NONE', #1200 ) ;
#2214=LINE ( 'NONE', #9435, #17096 ) ;
#2222=EDGE_CURVE ( 'NONE', #13428, #6792, #22485, .T. ) ;
#2229=ORIENTED_EDGE ( 'NONE', *, *, #7906, .T. ) ;
#2239=EDGE_LOOP ( 'NONE', ( #17435, #8425, #9225, #4011, #20545 ) ) ;
#2242=LINE ( 'NONE', #13281, #9188 ) ;
#2247=EDGE_LOOP ( 'NONE', ( #14580, #18347, #13625 ) ) ;
#2261=CARTESIAN_POINT ( 'NONE',  ( 24.75935218339999722, -28.32938697159999819, -147.5552959529999839 ) ) ;
#2262=PLANE ( 'NONE',  #18458 ) ;
#2267=ORIENTED_EDGE ( 'NONE', *, *, #9759, .T. ) ;
#2276=DIRECTION ( 'NONE',  ( 0.07970438983373200059, 0.9968185442904001770, -8.242295734823311485E-13 ) ) ;
#2281=FACE_OUTER_BOUND ( 'NONE', #7195, .T. ) ;
#2284=VERTEX_POINT ( 'NONE', #19026 ) ;
#2288=ORIENTED_EDGE ( 'NONE', *, *, #13914, .F. ) ;
#2289=AXIS2_PLACEMENT_3D ( 'NONE', #8985, #19840, #1532 ) ;
#2290=VECTOR ( 'NONE', #22504, 1000.000000000000227 ) ;
#2291=EDGE_LOOP ( 'NONE', ( #6808, #15232, #13159, #14299, #8994, #19423, #18000, #15179 ) ) ;
#2302=PLANE ( 'NONE',  #10309 ) ;
#2307=FACE_OUTER_BOUND ( 'NONE', #5624, .T. ) ;
#2312=ORIENTED_EDGE ( 'NONE', *, *, #13738, .T. ) ;
#2315=DIRECTION ( 'NONE',  ( -0.9919007982877544594, 0.1270149847699686418, 4.766005912188822159E-14 ) ) ;
#2316=ORIENTED_EDGE ( 'NONE', *, *, #12600, .T. ) ;
#2318=DIRECTION ( 'NONE',  ( -0.07970438983373200059, -0.9968185442904001770, 8.268133652483321323E-13 ) ) ;
#2324=AXIS2_PLACEMENT_3D ( 'NONE', #13079, #15231, #7950 ) ;
#2327=LINE ( 'NONE', #4092, #2595 ) ;
#2328=ORIENTED_EDGE ( 'NONE', *, *, #3849, .F. ) ;
#2337=VERTEX_POINT ( 'NONE', #2846 ) ;
#2350=ORIENTED_EDGE ( 'NONE', *, *, #15505, .T. ) ;
#2352=CIRCLE ( 'NONE', #11816, 5.999999999999998224 ) ;
#2353=VECTOR ( 'NONE', #1166, 1000.000000000000114 ) ;
#2354=ADVANCED_FACE ( 'NONE', ( #17353 ), #1068, .T. ) ;
#2358=EDGE_CURVE ( 'NONE', #8373, #12827, #5767, .T. ) ;
#2363=ORIENTED_EDGE ( 'NONE', *, *, #956, .F. ) ;
#2365=ORIENTED_EDGE ( 'NONE', *, *, #6046, .F. ) ;
#2387=CARTESIAN_POINT ( 'NONE',  ( 22.33963087269999903, -30.94765732060000119, -146.5552959529999839 ) ) ;
#2388=VERTEX_POINT ( 'NONE', #3877 ) ;
#2395=CARTESIAN_POINT ( 'NONE',  ( -9.157754307290000284, -15.75963164970000108, -147.5552959529999839 ) ) ;
#2397=CARTESIAN_POINT ( 'NONE',  ( 21.79964646190000011, -30.87346604779999737, -145.5552959529999839 ) ) ;
#2398=LINE ( 'NONE', #11172, #14153 ) ;
#2400=ORIENTED_EDGE ( 'NONE', *, *, #3159, .T. ) ;
#2407=AXIS2_PLACEMENT_3D ( 'NONE', #1642, #3177, #3645 ) ;
#2413=ORIENTED_EDGE ( 'NONE', *, *, #23486, .T. ) ;
#2416=EDGE_CURVE ( 'NONE', #7470, #5894, #5301, .T. ) ;
#2419=EDGE_CURVE ( 'NONE', #19198, #4115, #5647, .T. ) ;
#2427=EDGE_LOOP ( 'NONE', ( #7115, #6147, #20649, #23007 ) ) ;
#2436=ORIENTED_EDGE ( 'NONE', *, *, #15852, .F. ) ;
#2438=EDGE_CURVE ( 'NONE', #19256, #19447, #14586, .T. ) ;
#2439=FACE_OUTER_BOUND ( 'NONE', #8276, .T. ) ;
#2484=VECTOR ( 'NONE', #21541, 1000.000000000000114 ) ;
#2499=DIRECTION ( 'NONE',  ( -0.9949850929136110356, 0.1000233216789610247, -7.446425804567087094E-15 ) ) ;
#2506=VECTOR ( 'NONE', #7045, 1000.000000000000114 ) ;
#2508=AXIS2_PLACEMENT_3D ( 'NONE', #14330, #17666, #10499 ) ;
#2523=CARTESIAN_POINT ( 'NONE',  ( 8.633772787769999013, -29.00605602609999778, -147.5552959529999839 ) ) ;
#2533=EDGE_CURVE ( 'NONE', #17699, #13091, #2085, .T. ) ;
#2542=ORIENTED_EDGE ( 'NONE', *, *, #3842, .T. ) ;
#2544=PLANE ( 'NONE',  #4410 ) ;
#2550=ORIENTED_EDGE ( 'NONE', *, *, #13380, .F. ) ;
#2560=LINE ( 'NONE', #17417, #19780 ) ;
#2562=EDGE_CURVE ( 'NONE', #2284, #2706, #19153, .T. ) ;
#2567=EDGE_CURVE ( 'NONE', #5894, #1590, #22425, .T. ) ;
#2577=AXIS2_PLACEMENT_3D ( 'NONE', #69, #14579, #6516 ) ;
#2580=VERTEX_POINT ( 'NONE', #5994 ) ;
#2584=DIRECTION ( 'NONE',  ( 0.000000000000000000, 6.264364525598899972E-11, -1.000000000000000000 ) ) ;
#2585=ORIENTED_EDGE ( 'NONE', *, *, #14036, .F. ) ;
#2595=VECTOR ( 'NONE', #11326, 1000.000000000000000 ) ;
#2601=LINE ( 'NONE', #13298, #1208 ) ;
#2616=AXIS2_PLACEMENT_3D ( 'NONE', #16622, #7578, #14853 ) ;
#2618=VERTEX_POINT ( 'NONE', #5148 ) ;
#2619=CARTESIAN_POINT ( 'NONE',  ( 12.01554901919999985, -37.47280209340000567, -145.0552959529999839 ) ) ;
#2622=VERTEX_POINT ( 'NONE', #21357 ) ;
#2625=VECTOR ( 'NONE', #22025, 1000.000000000000000 ) ;
#2628=VERTEX_POINT ( 'NONE', #4809 ) ;
#2629=ORIENTED_EDGE ( 'NONE', *, *, #11125, .F. ) ;
#2630=DIRECTION ( 'NONE',  ( 1.000000000000000000, 0.000000000000000000, -8.953948693601887499E-12 ) ) ;
#2633=AXIS2_PLACEMENT_3D ( 'NONE', #18178, #17947, #8883 ) ;
#2635=LINE ( 'NONE', #20712, #22030 ) ;
#2639=AXIS2_PLACEMENT_3D ( 'NONE', #2619, #599, #7606 ) ;
#2645=EDGE_CURVE ( 'NONE', #2031, #1998, #3255, .T. ) ;
#2659=AXIS2_PLACEMENT_3D ( 'NONE', #8598, #14328, #6710 ) ;
#2661=LINE ( 'NONE', #4432, #22029 ) ;
#2664=DIRECTION ( 'NONE',  ( 2.839308199620000013E-14, 3.568879590630000244E-13, 1.000000000000000000 ) ) ;
#2666=CARTESIAN_POINT ( 'NONE',  ( 25.00000852249999994, -26.83294714660000224, -143.5552959529999839 ) ) ;
#2672=VECTOR ( 'NONE', #5152, 1000.000000000000000 ) ;
#2673=AXIS2_PLACEMENT_3D ( 'NONE', #21992, #7464, #12464 ) ;
#2680=CARTESIAN_POINT ( 'NONE',  ( -5.070907855429999778, -22.41528233759999722, -147.5552959529999839 ) ) ;
#2681=ORIENTED_EDGE ( 'NONE', *, *, #18120, .T. ) ;
#2700=VERTEX_POINT ( 'NONE', #8706 ) ;
#2706=VERTEX_POINT ( 'NONE', #22773 ) ;
#2711=DIRECTION ( 'NONE',  ( -0.9892101392001054760, 0.1465035852930155480, 4.471489433380478225E-12 ) ) ;
#2724=EDGE_CURVE ( 'NONE', #1140, #23501, #6701, .T. ) ;
#2729=FACE_OUTER_BOUND ( 'NONE', #12220, .T. ) ;
#2739=EDGE_LOOP ( 'NONE', ( #2798, #6479, #6612, #20977, #6785, #22477, #16616, #17206 ) ) ;
#2741=DIRECTION ( 'NONE',  ( 1.526468026909999897E-13, 8.159623473500000156E-13, 1.000000000000000000 ) ) ;
#2750=VERTEX_POINT ( 'NONE', #12175 ) ;
#2760=DIRECTION ( 'NONE',  ( -7.367827251323790032E-12, 0.000000000000000000, -1.000000000000000000 ) ) ;
#2763=DIRECTION ( 'NONE',  ( -0.9874789572432817186, 0.1577507813030449846, 2.479216961550704427E-14 ) ) ;
#2769=CARTESIAN_POINT ( 'NONE',  ( 7.228490359739999427, -13.33508289800000135, -146.5552959529999839 ) ) ;
#2775=EDGE_LOOP ( 'NONE', ( #836, #9835, #17267, #1204 ) ) ;
#2776=VECTOR ( 'NONE', #18591, 999.9999999999998863 ) ;
#2781=ADVANCED_FACE ( 'NONE', ( #9182 ), #14563, .F. ) ;
#2784=DIRECTION ( 'NONE',  ( -8.956391184260000029E-12, 9.094947017729999296E-13, -1.000000000000000000 ) ) ;
#2798=ORIENTED_EDGE ( 'NONE', *, *, #13125, .F. ) ;
#2806=ADVANCED_FACE ( 'NONE', ( #9292 ), #16565, .T. ) ;
#2809=ORIENTED_EDGE ( 'NONE', *, *, #7368, .F. ) ;
#2810=ORIENTED_EDGE ( 'NONE', *, *, #3283, .T. ) ;
#2813=VERTEX_POINT ( 'NONE', #7517 ) ;
#2816=ORIENTED_EDGE ( 'NONE', *, *, #14217, .T. ) ;
#2822=LINE ( 'NONE', #6734, #12933 ) ;
#2823=ADVANCED_FACE ( 'NONE', ( #275 ), #7172, .F. ) ;
#2831=CIRCLE ( 'NONE', #3974, 8.176568160360000448 ) ;
#2832=LINE ( 'NONE', #23495, #17755 ) ;
#2837=ORIENTED_EDGE ( 'NONE', *, *, #6869, .F. ) ;
#2840=ORIENTED_EDGE ( 'NONE', *, *, #4687, .T. ) ;
#2842=EDGE_CURVE ( 'NONE', #17230, #13656, #10408, .T. ) ;
#2843=LINE ( 'NONE', #17597, #14776 ) ;
#2845=EDGE_CURVE ( 'NONE', #22553, #22537, #13455, .T. ) ;
#2846=CARTESIAN_POINT ( 'NONE',  ( 19.75551406279999966, -31.14090339520000228, -145.5552959529999839 ) ) ;
#2852=VERTEX_POINT ( 'NONE', #22052 ) ;
#2865=CARTESIAN_POINT ( 'NONE',  ( -9.434278515689999978, -18.41834002140000237, -146.5552959529999839 ) ) ;
#2866=VERTEX_POINT ( 'NONE', #749 ) ;
#2871=CARTESIAN_POINT ( 'NONE',  ( 16.65421564080000039, -18.61497348660000029, -145.5552959529999839 ) ) ;
#2876=CARTESIAN_POINT ( 'NONE',  ( -9.363082409902974135, -24.97989489974943567, -147.5552959529923953 ) ) ;
#2877=LINE ( 'NONE', #3000, #6429 ) ;
#2879=DIRECTION ( 'NONE',  ( 8.954614827420000395E-12, -9.094947017729999296E-13, 1.000000000000000000 ) ) ;
#2894=VERTEX_POINT ( 'NONE', #7863 ) ;
#2896=CARTESIAN_POINT ( 'NONE',  ( 16.33424841169999908, -31.58611763329999889, -148.5552959529999839 ) ) ;
#2904=FILL_AREA_STYLE_COLOUR ( '', #22146 ) ;
#2909=VECTOR ( 'NONE', #15147, 1000.000000000000000 ) ;
#2927=EDGE_LOOP ( 'NONE', ( #19202, #2312, #18251, #1135, #8034 ) ) ;
#2929=VERTEX_POINT ( 'NONE', #13108 ) ;
#2950=VECTOR ( 'NONE', #13412, 999.9999999999998863 ) ;
#2951=CARTESIAN_POINT ( 'NONE',  ( 1.847645635000000119, -15.93876195360000025, -146.5552959529999839 ) ) ;
#2953=VECTOR ( 'NONE', #4150, 1000.000000000000114 ) ;
#2958=ORIENTED_EDGE ( 'NONE', *, *, #497, .T. ) ;
#2973=ADVANCED_FACE ( 'NONE', ( #6094 ), #18718, .T. ) ;
#2978=DIRECTION ( 'NONE',  ( -0.1270149847699686696, -0.9919007982877545704, 8.287421350277954308E-13 ) ) ;
#2982=DIRECTION ( 'NONE',  ( -0.9953753789357124848, 0.09606172499277225441, 7.355811845627876534E-14 ) ) ;
#2991=CARTESIAN_POINT ( 'NONE',  ( 5.347956485829999274, -22.34165470570000167, -146.5552959529999839 ) ) ;
#2993=DIRECTION ( 'NONE',  ( 1.526468026909999897E-13, 8.159623473500000156E-13, 1.000000000000000000 ) ) ;
#2994=EDGE_CURVE ( 'NONE', #4187, #11995, #12996, .T. ) ;
#2996=ORIENTED_EDGE ( 'NONE', *, *, #17303, .T. ) ;
#2998=ADVANCED_FACE ( 'NONE', ( #20270 ), #4074, .F. ) ;
#3000=CARTESIAN_POINT ( 'NONE',  ( 5.631397321050000571, -17.85059010000000157, -147.5552959529999839 ) ) ;
#3001=EDGE_CURVE ( 'NONE', #23414, #20938, #18469, .T. ) ;
#3003=CARTESIAN_POINT ( 'NONE',  ( -7.129475577410000042, -25.57825421080000083, -144.5552959529999839 ) ) ;
#3006=CARTESIAN_POINT ( 'NONE',  ( 23.17093239529999948, -15.44501179329999907, -144.0552959529999839 ) ) ;
#3009=ORIENTED_EDGE ( 'NONE', *, *, #12709, .F. ) ;
#3011=VECTOR ( 'NONE', #19976, 1000.000000000000000 ) ;
#3012=VECTOR ( 'NONE', #2784, 1000.000000000000000 ) ;
#3031=VECTOR ( 'NONE', #3216, 999.9999999999998863 ) ;
#3034=CARTESIAN_POINT ( 'NONE',  ( 6.830232017748067541, -28.71493780969095511, -144.5552959530278656 ) ) ;
#3043=LINE ( 'NONE', #22910, #10486 ) ;
#3052=EDGE_CURVE ( 'NONE', #20700, #18344, #20497, .T. ) ;
#3054=VECTOR ( 'NONE', #12463, 999.9999999999998863 ) ;
#3058=ORIENTED_EDGE ( 'NONE', *, *, #3585, .F. ) ;
#3059=EDGE_LOOP ( 'NONE', ( #561, #7030, #15212, #3298, #21693, #7616 ) ) ;
#3062=CARTESIAN_POINT ( 'NONE',  ( 4.374398326270000581, -26.09174856970000178, -143.5552959529999839 ) ) ;
#3065=CARTESIAN_POINT ( 'NONE',  ( -6.603585321229999749, -20.59801339440000234, -143.5552959529999839 ) ) ;
#3068=VECTOR ( 'NONE', #2276, 1000.000000000000114 ) ;
#3080=EDGE_CURVE ( 'NONE', #11246, #20820, #12262, .T. ) ;
#3095=FACE_OUTER_BOUND ( 'NONE', #7603, .T. ) ;
#3097=AXIS2_PLACEMENT_3D ( 'NONE', #14363, #8756, #16035 ) ;
#3102=FACE_OUTER_BOUND ( 'NONE', #4595, .T. ) ;
#3115=VERTEX_POINT ( 'NONE', #8563 ) ;
#3116=AXIS2_PLACEMENT_3D ( 'NONE', #15395, #10140, #10272 ) ;
#3132=AXIS2_PLACEMENT_3D ( 'NONE', #11251, #18766, #18523 ) ;
#3134=EDGE_CURVE ( 'NONE', #21766, #5773, #23101, .T. ) ;
#3144=CARTESIAN_POINT ( 'NONE',  ( 20.58976242830000203, -31.80400447969999789, -143.5552959529999839 ) ) ;
#3145=EDGE_CURVE ( 'NONE', #18669, #3418, #20976, .T. ) ;
#3148=PLANE ( 'NONE',  #23254 ) ;
#3154=CARTESIAN_POINT ( 'NONE',  ( 23.08797222880000177, -15.45109671570000032, -143.0552959529999839 ) ) ;
#3157=EDGE_CURVE ( 'NONE', #18609, #20700, #8334, .T. ) ;
#3159=EDGE_CURVE ( 'NONE', #1590, #1140, #22873, .T. ) ;
#3165=CARTESIAN_POINT ( 'NONE',  ( -4.946601369560000627, -23.77962690289999870, -144.0552959529999839 ) ) ;
#3166=DIRECTION ( 'NONE',  ( 0.1985297072190585210, 0.9800948705872890576, -8.351208274002460500E-13 ) ) ;
#3169=EDGE_LOOP ( 'NONE', ( #1224, #11127, #9310 ) ) ;
#3170=EDGE_LOOP ( 'NONE', ( #22135, #900, #9249, #17936, #11292 ) ) ;
#3177=DIRECTION ( 'NONE',  ( 4.430318231639999944E-12, -6.100259101500000139E-13, 1.000000000000000000 ) ) ;
#3180=CARTESIAN_POINT ( 'NONE',  ( 24.85988213910000155, -26.16224997189999968, -145.5552959529999839 ) ) ;
#3195=ORIENTED_EDGE ( 'NONE', *, *, #7805, .F. ) ;
#3202=CARTESIAN_POINT ( 'NONE',  ( -9.434278515689999978, -18.41834002140000237, -146.5552959529999839 ) ) ;
#3204=FACE_OUTER_BOUND ( 'NONE', #19712, .T. ) ;
#3216=DIRECTION ( 'NONE',  ( -0.9954742291034677226, 0.09503188512734457583, 4.503363594322118746E-12 ) ) ;
#3226=CARTESIAN_POINT ( 'NONE',  ( -8.296392858609999976, -9.821782169089999570, -148.5552959529999839 ) ) ;
#3229=CARTESIAN_POINT ( 'NONE',  ( 1.591914056710000080, -18.48847405160000079, -143.5552959529999839 ) ) ;
#3238=ORIENTED_EDGE ( 'NONE', *, *, #7901, .T. ) ;
#3246=DIRECTION ( 'NONE',  ( -0.2208456705930775810, -0.9753087663813413410, 1.089717887850382194E-12 ) ) ;
#3255=LINE ( 'NONE', #15637, #7386 ) ;
#3257=DIRECTION ( 'NONE',  ( 1.000000000000000000, 0.000000000000000000, -4.431640239962082113E-12 ) ) ;
#3261=ORIENTED_EDGE ( 'NONE', *, *, #3666, .F. ) ;
#3266=FACE_OUTER_BOUND ( 'NONE', #9472, .T. ) ;
#3267=ADVANCED_FACE ( 'NONE', ( #12732 ), #9156, .T. ) ;
#3271=FACE_OUTER_BOUND ( 'NONE', #10038, .T. ) ;
#3275=AXIS2_PLACEMENT_3D ( 'NONE', #3625, #9194, #173 ) ;
#3278=EDGE_CURVE ( 'NONE', #4889, #10478, #6914, .T. ) ;
#3283=EDGE_CURVE ( 'NONE', #19376, #1427, #18340, .T. ) ;
#3286=EDGE_CURVE ( 'NONE', #30, #22422, #2831, .T. ) ;
#3297=CARTESIAN_POINT ( 'NONE',  ( 5.792747474889999637, -16.92794981449999980, -144.5552959529999839 ) ) ;
#3298=ORIENTED_EDGE ( 'NONE', *, *, #8919, .T. ) ;
#3304=ORIENTED_EDGE ( 'NONE', *, *, #6206, .T. ) ;
#3305=LINE ( 'NONE', #1658, #10696 ) ;
#3308=EDGE_CURVE ( 'NONE', #8795, #9023, #20124, .T. ) ;
#3311=ORIENTED_EDGE ( 'NONE', *, *, #20813, .F. ) ;
#3313=ORIENTED_EDGE ( 'NONE', *, *, #3080, .T. ) ;
#3314=LINE ( 'NONE', #14505, #11352 ) ;
#3318=CARTESIAN_POINT ( 'NONE',  ( -4.021770264099999714, -29.17051924670000318, -143.5552959529999839 ) ) ;
#3323=ORIENTED_EDGE ( 'NONE', *, *, #20640, .T. ) ;
#3329=LINE ( 'NONE', #23439, #6744 ) ;
#3340=DIRECTION ( 'NONE',  ( -1.526468026909999897E-13, -8.159623473500000156E-13, -1.000000000000000000 ) ) ;
#3344=DIRECTION ( 'NONE',  ( -1.525446435830000185E-13, -8.171241461240000022E-13, -1.000000000000000000 ) ) ;
#3346=DIRECTION ( 'NONE',  ( 0.1000233216789610108, 0.9949850929136109245, -3.588240815588595806E-13 ) ) ;
#3348=ORIENTED_EDGE ( 'NONE', *, *, #5333, .T. ) ;
#3349=DIRECTION ( 'NONE',  ( 1.000000000000000000, 0.000000000000000000, -4.431640239962082113E-12 ) ) ;
#3350=EDGE_LOOP ( 'NONE', ( #19538, #6492, #10581 ) ) ;
#3363=ORIENTED_EDGE ( 'NONE', *, *, #13746, .T. ) ;
#3368=CARTESIAN_POINT ( 'NONE',  ( -9.347107914279998653, -17.32706600430000066, -143.5552959529999839 ) ) ;
#3369=DIRECTION ( 'NONE',  ( 1.526468026909999897E-13, 8.159623473500000156E-13, 1.000000000000000000 ) ) ;
#3370=DIRECTION ( 'NONE',  ( -0.9954742291034676116, 0.09503188512734456195, 0.000000000000000000 ) ) ;
#3373=DIRECTION ( 'NONE',  ( 4.430318231639999944E-12, -6.100259101500000139E-13, 1.000000000000000000 ) ) ;
#3379=VECTOR ( 'NONE', #4751, 1000.000000000000000 ) ;
#3383=PLANE ( 'NONE',  #23080 ) ;
#3386=AXIS2_PLACEMENT_3D ( 'NONE', #7523, #1966, #14677 ) ;
#3402=PLANE ( 'NONE',  #2407 ) ;
#3404=ORIENTED_EDGE ( 'NONE', *, *, #10243, .T. ) ;
#3406=CIRCLE ( 'NONE', #2289, 5.000000000000000000 ) ;
#3413=LINE ( 'NONE', #14359, #21256 ) ;
#3414=AXIS2_PLACEMENT_3D ( 'NONE', #1800, #11162, #4039 ) ;
#3418=VERTEX_POINT ( 'NONE', #9729 ) ;
#3425=ORIENTED_EDGE ( 'NONE', *, *, #23166, .T. ) ;
#3432=AXIS2_PLACEMENT_3D ( 'NONE', #3989, #13378, #7778 ) ;
#3434=AXIS2_PLACEMENT_3D ( 'NONE', #3970, #16814, #5859 ) ;
#3442=DIRECTION ( 'NONE',  ( 2.839308199620000013E-14, 3.568879590630000244E-13, 1.000000000000000000 ) ) ;
#3443=EDGE_LOOP ( 'NONE', ( #7897, #4712, #9612, #19932, #9943, #22634 ) ) ;
#3446=EDGE_CURVE ( 'NONE', #20874, #3831, #1909, .T. ) ;
#3447=EDGE_LOOP ( 'NONE', ( #8988, #4145, #18435, #19444, #19650, #22907, #18617 ) ) ;
#3456=DIRECTION ( 'NONE',  ( -0.9840552701943220404, 0.1778629393740580045, -3.541738516501160129E-14 ) ) ;
#3457=DIRECTION ( 'NONE',  ( 1.526468026909999897E-13, 8.159623473500000156E-13, 1.000000000000000000 ) ) ;
#3458=FACE_OUTER_BOUND ( 'NONE', #12852, .T. ) ;
#3470=LINE ( 'NONE', #10707, #9434 ) ;
#3479=DIRECTION ( 'NONE',  ( -0.9954742291034677226, 0.09503188512734457583, 4.502513436702118395E-12 ) ) ;
#3490=DIRECTION ( 'NONE',  ( -0.8319143897030502055, -0.5549039990890329843, 3.347322419244847777E-12 ) ) ;
#3493=LINE ( 'NONE', #12396, #17938 ) ;
#3496=ORIENTED_EDGE ( 'NONE', *, *, #1252, .F. ) ;
#3497=LINE ( 'NONE', #5051, #14440 ) ;
#3499=AXIS2_PLACEMENT_3D ( 'NONE', #11982, #9959, #20808 ) ;
#3501=ORIENTED_EDGE ( 'NONE', *, *, #3717, .F. ) ;
#3502=EDGE_CURVE ( 'NONE', #4852, #22736, #22796, .T. ) ;
#3503=AXIS2_PLACEMENT_3D ( 'NONE', #12520, #21824, #18125 ) ;
#3508=ADVANCED_FACE ( 'NONE', ( #7955 ), #14991, .T. ) ;
#3510=CARTESIAN_POINT ( 'NONE',  ( -9.969904307360000217, -22.67446893780000039, -145.0552959529999839 ) ) ;
#3516=ORIENTED_EDGE ( 'NONE', *, *, #20975, .T. ) ;
#3526=CARTESIAN_POINT ( 'NONE',  ( 23.99773978629999860, -29.25880395889999974, -147.5552959529999839 ) ) ;
#3534=VERTEX_POINT ( 'NONE', #12114 ) ;
#3544=ORIENTED_EDGE ( 'NONE', *, *, #1462, .T. ) ;
#3549=ORIENTED_EDGE ( 'NONE', *, *, #23043, .F. ) ;
#3555=EDGE_CURVE ( 'NONE', #1038, #22422, #4868, .T. ) ;
#3558=CARTESIAN_POINT ( 'NONE',  ( 7.228490359739999427, -13.33508289800000135, -145.5552959529999839 ) ) ;
#3561=CARTESIAN_POINT ( 'NONE',  ( 16.16922456049999823, -22.27514461170000004, -147.5552959529999839 ) ) ;
#3565=EDGE_CURVE ( 'NONE', #16716, #18274, #8073, .T. ) ;
#3584=CARTESIAN_POINT ( 'NONE',  ( -6.072796602490000417, -14.62912504250000012, -144.5552959529999839 ) ) ;
#3585=EDGE_CURVE ( 'NONE', #5977, #21733, #22964, .T. ) ;
#3601=DIRECTION ( 'NONE',  ( 0.9985681355238719137, -0.05349466063429310358, -4.511742413209420161E-12 ) ) ;
#3611=ADVANCED_FACE ( 'NONE', ( #11997 ), #11879, .T. ) ;
#3613=PLANE ( 'NONE',  #19072 ) ;
#3618=CARTESIAN_POINT ( 'NONE',  ( -9.334216945200001447, -17.19633444960000190, -146.5552959529999839 ) ) ;
#3624=CARTESIAN_POINT ( 'NONE',  ( -6.603585321229999749, -20.59801339440000234, -143.5552959529999839 ) ) ;
#3625=CARTESIAN_POINT ( 'NONE',  ( 23.50000000000000000, -20.50000000000000000, -144.7152959530000089 ) ) ;
#3630=CARTESIAN_POINT ( 'NONE',  ( 16.65421564080000039, -18.61497348660000029, -145.5552959529999839 ) ) ;
#3645=DIRECTION ( 'NONE',  ( 1.000000000000000000, 0.000000000000000000, -4.430318231639999944E-12 ) ) ;
#3649=ORIENTED_EDGE ( 'NONE', *, *, #744, .F. ) ;
#3652=VECTOR ( 'NONE', #15946, 1000.000000000000227 ) ;
#3655=ORIENTED_EDGE ( 'NONE', *, *, #3663, .F. ) ;
#3663=EDGE_CURVE ( 'NONE', #23456, #19736, #6295, .T. ) ;
#3666=EDGE_CURVE ( 'NONE', #6279, #14794, #11753, .T. ) ;
#3674=CARTESIAN_POINT ( 'NONE',  ( 2.170391987449999505, -12.72823260819999902, -145.5552959529999839 ) ) ;
#3675=LINE ( 'NONE', #3561, #9103 ) ;
#3676=DIRECTION ( 'NONE',  ( 1.000000000000000000, 0.000000000000000000, -2.715621035259064790E-14 ) ) ;
#3682=EDGE_CURVE ( 'NONE', #11025, #19591, #20522, .T. ) ;
#3687=ORIENTED_EDGE ( 'NONE', *, *, #2358, .F. ) ;
#3689=DIRECTION ( 'NONE',  ( 4.510170015240000199E-12, -1.314504061159999897E-13, 1.000000000000000000 ) ) ;
#3690=DIRECTION ( 'NONE',  ( -0.9954742291034677226, 0.09503188512734457583, 4.503697062742119365E-12 ) ) ;
#3700=AXIS2_PLACEMENT_3D ( 'NONE', #10858, #14454, #15765 ) ;
#3717=EDGE_CURVE ( 'NONE', #23501, #4187, #21774, .T. ) ;
#3725=DIRECTION ( 'NONE',  ( 0.000000000000000000, -1.000000000000000000, 8.159623473500000156E-13 ) ) ;
#3726=DIRECTION ( 'NONE',  ( 1.000000000000000000, 0.000000000000000000, -4.510774274160000731E-12 ) ) ;
#3731=ORIENTED_EDGE ( 'NONE', *, *, #50, .T. ) ;
#3733=VECTOR ( 'NONE', #23240, 1000.000000000000000 ) ;
#3734=PLANE ( 'NONE',  #3386 ) ;
#3737=LINE ( 'NONE', #3624, #17874 ) ;
#3738=ADVANCED_FACE ( 'NONE', ( #3204 ), #5459, .T. ) ;
#3739=DIRECTION ( 'NONE',  ( 4.430233957459999899E-12, -6.110667527539999876E-13, 1.000000000000000000 ) ) ;
#3740=EDGE_CURVE ( 'NONE', #3831, #10198, #19390, .T. ) ;
#3748=ORIENTED_EDGE ( 'NONE', *, *, #20592, .T. ) ;
#3749=VECTOR ( 'NONE', #13637, 1000.000000000000227 ) ;
#3755=DIRECTION ( 'NONE',  ( 0.2451800884060535979, 0.9694775522152123681, -1.317373699560290683E-12 ) ) ;
#3761=ORIENTED_EDGE ( 'NONE', *, *, #3502, .F. ) ;
#3769=EDGE_CURVE ( 'NONE', #7769, #20668, #5344, .T. ) ;
#3772=AXIS2_PLACEMENT_3D ( 'NONE', #8330, #3340, #10577 ) ;
#3778=ORIENTED_EDGE ( 'NONE', *, *, #11258, .T. ) ;
#3784=PRODUCT_CONTEXT ( 'NONE', #9918, 'mechanical' ) ;
#3800=DIRECTION ( 'NONE',  ( 4.430233957459999899E-12, -6.110667527539999876E-13, 1.000000000000000000 ) ) ;
#3810=VECTOR ( 'NONE', #7889, 1000.000000000000000 ) ;
#3814=DIRECTION ( 'NONE',  ( 8.955190032050000935E-12, -9.104778821549999739E-13, 1.000000000000000000 ) ) ;
#3815=AXIS2_PLACEMENT_3D ( 'NONE', #10620, #1497, #12184 ) ;
#3816=DIRECTION ( 'NONE',  ( 8.955190032050000935E-12, -9.104778821549999739E-13, 1.000000000000000000 ) ) ;
#3818=ORIENTED_EDGE ( 'NONE', *, *, #9759, .F. ) ;
#3821=DIRECTION ( 'NONE',  ( -1.769477252542410170E-11, 0.000000000000000000, 1.000000000000000000 ) ) ;
#3825=LINE ( 'NONE', #7274, #2625 ) ;
#3826=DIRECTION ( 'NONE',  ( 0.000000000000000000, -1.000000000000000000, 8.159623473500000156E-13 ) ) ;
#3827=ORIENTED_EDGE ( 'NONE', *, *, #14838, .T. ) ;
#3829=AXIS2_PLACEMENT_3D ( 'NONE', #7095, #1874, #16382 ) ;
#3831=VERTEX_POINT ( 'NONE', #19972 ) ;
#3835=CYLINDRICAL_SURFACE ( 'NONE', #12518, 5.999999999999999112 ) ;
#3837=CARTESIAN_POINT ( 'NONE',  ( 24.59017985859999911, -26.91621017459999976, -147.5552959529999839 ) ) ;
#3840=FACE_OUTER_BOUND ( 'NONE', #10713, .T. ) ;
#3842=EDGE_CURVE ( 'NONE', #2622, #1486, #16287, .T. ) ;
#3849=EDGE_CURVE ( 'NONE', #17357, #22329, #1428, .T. ) ;
#3852=EDGE_LOOP ( 'NONE', ( #16503, #2413, #5372, #21942 ) ) ;
#3855=CARTESIAN_POINT ( 'NONE',  ( -6.049191701419999845, -14.51144913589999952, -146.5552959529999839 ) ) ;
#3876=CIRCLE ( 'NONE', #3116, 2.999999999999999112 ) ;
#3877=CARTESIAN_POINT ( 'NONE',  ( 23.08797222880000177, -15.45109671570000032, -143.5552959529999839 ) ) ;
#3886=EDGE_LOOP ( 'NONE', ( #1726, #4484, #8733, #18407, #18045 ) ) ;
#3894=VECTOR ( 'NONE', #2879, 1000.000000000000000 ) ;
#3895=VECTOR ( 'NONE', #17954, 1000.000000000000114 ) ;
#3908=DIRECTION ( 'NONE',  ( 1.527666881879999979E-13, 8.171241461240000022E-13, 1.000000000000000000 ) ) ;
#3909=EDGE_CURVE ( 'NONE', #13656, #18172, #15901, .T. ) ;
#3913=AXIS2_PLACEMENT_3D ( 'NONE', #8565, #15837, #23103 ) ;
#3914=PLANE ( 'NONE',  #10248 ) ;
#3920=DIRECTION ( 'NONE',  ( -0.09606172499277226828, -0.9953753789357124848, 8.268133652477615271E-13 ) ) ;
#3950=CARTESIAN_POINT ( 'NONE',  ( 15.59498359470000040, -26.23371093219999750, -147.5552959529999839 ) ) ;
#3955=CARTESIAN_POINT ( 'NONE',  ( 24.11847952820000174, -31.58456057200000089, -142.5552959529999839 ) ) ;
#3960=VECTOR ( 'NONE', #15134, 1000.000000000000227 ) ;
#3963=EDGE_CURVE ( 'NONE', #7923, #13663, #18767, .T. ) ;
#3964=CARTESIAN_POINT ( 'NONE',  ( 1.342750202250000191, -63.28208324180000233, -144.0552959529999839 ) ) ;
#3967=ORIENTED_EDGE ( 'NONE', *, *, #18531, .T. ) ;
#3970=CARTESIAN_POINT ( 'NONE',  ( 21.44117969379999877, -21.36894679869999791, -146.5552959529999839 ) ) ;
#3971=ORIENTED_EDGE ( 'NONE', *, *, #4430, .T. ) ;
#3974=AXIS2_PLACEMENT_3D ( 'NONE', #14177, #18219, #21442 ) ;
#3975=DIRECTION ( 'NONE',  ( 0.9953753789357124848, -0.09606172499277225441, -7.355811845627870223E-14 ) ) ;
#3989=CARTESIAN_POINT ( 'NONE',  ( 23.49999999970000175, -20.50000000000000000, -148.5552959529999839 ) ) ;
#3993=ORIENTED_EDGE ( 'NONE', *, *, #11131, .F. ) ;
#3995=EDGE_CURVE ( 'NONE', #6018, #5559, #689, .T. ) ;
#4002=ADVANCED_FACE ( 'NONE', ( #2128 ), #9349, .T. ) ;
#4003=EDGE_CURVE ( 'NONE', #4587, #11453, #6379, .T. ) ;
#4011=ORIENTED_EDGE ( 'NONE', *, *, #18752, .F. ) ;
#4016=ORIENTED_EDGE ( 'NONE', *, *, #2099, .T. ) ;
#4017=SHAPE_DEFINITION_REPRESENTATION ( #16047, #15746 ) ;
#4032=EDGE_CURVE ( 'NONE', #1892, #15749, #20915, .T. ) ;
#4034=DIRECTION ( 'NONE',  ( 8.955190032049260996E-12, -9.104778821548929412E-13, 1.000000000000000000 ) ) ;
#4039=DIRECTION ( 'NONE',  ( 1.000000000000000000, 0.000000000000000000, -4.510774274160000731E-12 ) ) ;
#4041=PLANE ( 'NONE',  #6784 ) ;
#4042=AXIS2_PLACEMENT_3D ( 'NONE', #17368, #13683, #2630 ) ;
#4049=FACE_OUTER_BOUND ( 'NONE', #14988, .T. ) ;
#4054=CARTESIAN_POINT ( 'NONE',  ( -4.021770264099999714, -29.17051924670000318, -142.5552959529999839 ) ) ;
#4066=LINE ( 'NONE', #20489, #15883 ) ;
#4070=VECTOR ( 'NONE', #19576, 1000.000000000000000 ) ;
#4074=CYLINDRICAL_SURFACE ( 'NONE', #923, 35.00000000000000000 ) ;
#4077=DIRECTION ( 'NONE',  ( 1.000000000000000000, 0.000000000000000000, -1.522591576628786004E-13 ) ) ;
#4089=CARTESIAN_POINT ( 'NONE',  ( 4.374398326270000581, -26.09174856970000178, -144.5552959529999839 ) ) ;
#4092=CARTESIAN_POINT ( 'NONE',  ( 20.31210873290000052, -31.32069079449999904, -147.0552959529999839 ) ) ;
#4098=PLANE ( 'NONE',  #16034 ) ;
#4101=DIRECTION ( 'NONE',  ( 1.000000000000000000, 0.000000000000000000, -2.775557561562892298E-14 ) ) ;
#4115=VERTEX_POINT ( 'NONE', #15319 ) ;
#4119=ORIENTED_EDGE ( 'NONE', *, *, #7673, .F. ) ;
#4120=CYLINDRICAL_SURFACE ( 'NONE', #9822, 5.999999999999999112 ) ;
#4122=EDGE_LOOP ( 'NONE', ( #20523, #16555, #6073, #5554 ) ) ;
#4123=PLANE ( 'NONE',  #6839 ) ;
#4124=ORIENTED_EDGE ( 'NONE', *, *, #16868, .T. ) ;
#4128=CARTESIAN_POINT ( 'NONE',  ( -5.070907855439999778, -22.41528233759999722, -148.5552959529999839 ) ) ;
#4133=EDGE_CURVE ( 'NONE', #17961, #7102, #8402, .T. ) ;
#4145=ORIENTED_EDGE ( 'NONE', *, *, #10917, .T. ) ;
#4150=DIRECTION ( 'NONE',  ( -0.07970438983373200059, -0.9968185442904001770, 8.268372250843320857E-13 ) ) ;
#4155=DIRECTION ( 'NONE',  ( 1.000000000000000000, 0.000000000000000000, -8.955799065309598247E-12 ) ) ;
#4157=LINE ( 'NONE', #22015, #4888 ) ;
#4169=DIRECTION ( 'NONE',  ( 0.4144957952930628520, -0.9100512269561374934, 6.800116025829078761E-13 ) ) ;
#4171=ADVANCED_FACE ( 'NONE', ( #4962 ), #21503, .F. ) ;
#4175=ORIENTED_EDGE ( 'NONE', *, *, #21775, .F. ) ;
#4180=AXIS2_PLACEMENT_3D ( 'NONE', #19676, #3373, #3257 ) ;
#4187=VERTEX_POINT ( 'NONE', #14122 ) ;
#4188=FACE_OUTER_BOUND ( 'NONE', #11119, .T. ) ;
#4189=DIRECTION ( 'NONE',  ( -2.842170943040000002E-14, -3.570477247189999985E-13, -1.000000000000000000 ) ) ;
#4197=CARTESIAN_POINT ( 'NONE',  ( 1.354168148130000082, -20.95195702430000040, -144.0552959529999839 ) ) ;
#4203=CARTESIAN_POINT ( 'NONE',  ( 7.085709294149999060, -13.66851965709999916, -143.5552959529999839 ) ) ;
#4208=DIRECTION ( 'NONE',  ( 0.9944529286486341046, -0.1051825684329612265, -4.469111776238355154E-12 ) ) ;
#4212=CARTESIAN_POINT ( 'NONE',  ( -9.282104535849999394, -16.71402168319999859, -144.5552959529999839 ) ) ;
#4216=ORIENTED_EDGE ( 'NONE', *, *, #18880, .T. ) ;
#4219=ADVANCED_FACE ( 'NONE', ( #7093 ), #9096, .F. ) ;
#4225=ORIENTED_EDGE ( 'NONE', *, *, #11237, .F. ) ;
#4231=CIRCLE ( 'NONE', #23239, 8.176568160359998672 ) ;
#4237=ORIENTED_EDGE ( 'NONE', *, *, #8774, .T. ) ;
#4238=FACE_OUTER_BOUND ( 'NONE', #1795, .T. ) ;
#4240=LINE ( 'NONE', #914, #12844 ) ;
#4249=ORIENTED_EDGE ( 'NONE', *, *, #15459, .T. ) ;
#4255=DIRECTION ( 'NONE',  ( -8.955190032050000935E-12, 9.104778821549999739E-13, -1.000000000000000000 ) ) ;
#4261=CIRCLE ( 'NONE', #11460, 6.000000000000001776 ) ;
#4266=DIRECTION ( 'NONE',  ( -0.9954742291034677226, 0.09503188512734457583, 4.502513436702118395E-12 ) ) ;
#4277=CARTESIAN_POINT ( 'NONE',  ( 16.64676602990000021, -18.64223989710000140, -144.0552959529999839 ) ) ;
#4279=CARTESIAN_POINT ( 'NONE',  ( 4.468795199060000556, -26.40504320680000205, -143.5552959529999839 ) ) ;
#4293=CARTESIAN_POINT ( 'NONE',  ( 23.78818517497831664, -17.51387386319286321, -144.7152959530024816 ) ) ;
#4294=ORIENTED_EDGE ( 'NONE', *, *, #13716, .T. ) ;
#4298=FACE_OUTER_BOUND ( 'NONE', #17298, .T. ) ;
#4305=DIRECTION ( 'NONE',  ( -0.9874789572432817186, 0.1577507813030449846, 2.191150709840624368E-14 ) ) ;
#4308=ADVANCED_FACE ( 'NONE', ( #13578 ), #13031, .T. ) ;
#4310=ADVANCED_FACE ( 'NONE', ( #11003 ), #9216, .F. ) ;
#4329=CARTESIAN_POINT ( 'NONE',  ( -6.072796602490000417, -14.62912504250000012, -144.0552959529999839 ) ) ;
#4342=ORIENTED_EDGE ( 'NONE', *, *, #3446, .T. ) ;
#4351=EDGE_CURVE ( 'NONE', #473, #9406, #20731, .T. ) ;
#4353=ORIENTED_EDGE ( 'NONE', *, *, #11404, .F. ) ;
#4357=CARTESIAN_POINT ( 'NONE',  ( -4.959431410700000598, -23.66636161550000139, -146.5552959529999839 ) ) ;
#4380=LINE ( 'NONE', #22238, #2153 ) ;
#4385=DIRECTION ( 'NONE',  ( 0.000000000000000000, -1.000000000000000000, 8.159623473500000156E-13 ) ) ;
#4392=VECTOR ( 'NONE', #9744, 999.9999999999998863 ) ;
#4394=ORIENTED_EDGE ( 'NONE', *, *, #11852, .F. ) ;
#4397=ORIENTED_EDGE ( 'NONE', *, *, #109, .F. ) ;
#4408=DIRECTION ( 'NONE',  ( 1.000000000000000000, 0.000000000000000000, -4.510774274160000731E-12 ) ) ;
#4410=AXIS2_PLACEMENT_3D ( 'NONE', #15383, #2664, #16818 ) ;
#4424=DIRECTION ( 'NONE',  ( -1.526468026909999897E-13, -8.159623473500000156E-13, -1.000000000000000000 ) ) ;
#4430=EDGE_CURVE ( 'NONE', #1380, #11626, #23227, .T. ) ;
#4432=CARTESIAN_POINT ( 'NONE',  ( -9.056357402059999728, -12.43025388040000045, -147.0552959529999839 ) ) ;
#4433=ORIENTED_EDGE ( 'NONE', *, *, #5957, .T. ) ;
#4450=CARTESIAN_POINT ( 'NONE',  ( -9.873006318519999880, -23.84776512999999909, -143.5552959529999839 ) ) ;
#4466=ORIENTED_EDGE ( 'NONE', *, *, #21477, .T. ) ;
#4467=DIRECTION ( 'NONE',  ( 1.526468026909999897E-13, 8.159623473500000156E-13, 1.000000000000000000 ) ) ;
#4473=CARTESIAN_POINT ( 'NONE',  ( -10.01911575600000148, -21.69748113039999637, -148.5552959529999839 ) ) ;
#4484=ORIENTED_EDGE ( 'NONE', *, *, #23188, .F. ) ;
#4506=VECTOR ( 'NONE', #11252, 1000.000000000000000 ) ;
#4511=ORIENTED_EDGE ( 'NONE', *, *, #7438, .F. ) ;
#4520=ORIENTED_EDGE ( 'NONE', *, *, #15459, .F. ) ;
#4529=DIRECTION ( 'NONE',  ( 4.510774274160000731E-12, -1.321907670990000086E-13, 1.000000000000000000 ) ) ;
#4539=CARTESIAN_POINT ( 'NONE',  ( -9.157754307290000284, -15.75963164970000108, -147.5552959529999839 ) ) ;
#4564=VERTEX_POINT ( 'NONE', #14650 ) ;
#4568=VECTOR ( 'NONE', #5334, 1000.000000000000114 ) ;
#4572=ADVANCED_FACE ( 'NONE', ( #5600 ), #20127, .F. ) ;
#4576=ORIENTED_EDGE ( 'NONE', *, *, #7493, .T. ) ;
#4587=VERTEX_POINT ( 'NONE', #5374 ) ;
#4589=ORIENTED_EDGE ( 'NONE', *, *, #22294, .T. ) ;
#4590=CARTESIAN_POINT ( 'NONE',  ( 0.000000000000000000, 0.000000000000000000, 0.000000000000000000 ) ) ;
#4591=EDGE_CURVE ( 'NONE', #919, #8980, #257, .T. ) ;
#4593=LINE ( 'NONE', #17319, #22016 ) ;
#4595=EDGE_LOOP ( 'NONE', ( #19373, #6293, #12167, #18832 ) ) ;
#4598=VERTEX_POINT ( 'NONE', #8810 ) ;
#4614=VECTOR ( 'NONE', #16072, 1000.000000000000114 ) ;
#4619=VERTEX_POINT ( 'NONE', #7150 ) ;
#4625=ORIENTED_EDGE ( 'NONE', *, *, #819, .F. ) ;
#4628=ADVANCED_FACE ( 'NONE', ( #14415 ), #7032, .T. ) ;
#4638=VECTOR ( 'NONE', #18546, 1000.000000000000000 ) ;
#4648=DIRECTION ( 'NONE',  ( -0.9938526945756315234, 0.1107105301439589573, 0.000000000000000000 ) ) ;
#4657=EDGE_CURVE ( 'NONE', #10198, #15664, #9032, .T. ) ;
#4662=FACE_OUTER_BOUND ( 'NONE', #5527, .T. ) ;
#4663=FACE_OUTER_BOUND ( 'NONE', #6718, .T. ) ;
#4672=CIRCLE ( 'NONE', #1649, 35.00000000000000000 ) ;
#4682=DIRECTION ( 'NONE',  ( -1.527666881879999979E-13, -8.153477892850000134E-13, -1.000000000000000000 ) ) ;
#4687=EDGE_CURVE ( 'NONE', #23020, #5244, #11289, .T. ) ;
#4689=ORIENTED_EDGE ( 'NONE', *, *, #6298, .T. ) ;
#4695=DIRECTION ( 'NONE',  ( 1.526468026909999897E-13, 8.159623473500000156E-13, 1.000000000000000000 ) ) ;
#4706=VERTEX_POINT ( 'NONE', #9733 ) ;
#4707=PLANE ( 'NONE',  #22344 ) ;
#4708=EDGE_CURVE ( 'NONE', #19961, #22823, #14996, .T. ) ;
#4711=DIRECTION ( 'NONE',  ( 0.9999976651796518290, -0.002160933882609249439, -8.955304954746877373E-12 ) ) ;
#4712=ORIENTED_EDGE ( 'NONE', *, *, #4133, .T. ) ;
#4716=AXIS2_PLACEMENT_3D ( 'NONE', #17031, #11544, #9405 ) ;
#4724=FACE_OUTER_BOUND ( 'NONE', #6257, .T. ) ;
#4729=ORIENTED_EDGE ( 'NONE', *, *, #11781, .T. ) ;
#4740=EDGE_LOOP ( 'NONE', ( #14376, #15588, #9277, #4874, #16642, #930, #11341 ) ) ;
#4747=CYLINDRICAL_SURFACE ( 'NONE', #16812, 35.00000000000000000 ) ;
#4751=DIRECTION ( 'NONE',  ( 4.430233957459999899E-12, -6.110667527539999876E-13, 1.000000000000000000 ) ) ;
#4754=VERTEX_POINT ( 'NONE', #4054 ) ;
#4769=DIRECTION ( 'NONE',  ( 4.510774274160000731E-12, -1.321907670990000086E-13, 1.000000000000000000 ) ) ;
#4781=LINE ( 'NONE', #3006, #20519 ) ;
#4793=DIRECTION ( 'NONE',  ( 1.000000000000000000, 0.000000000000000000, -4.511206223393553012E-12 ) ) ;
#4801=ORIENTED_EDGE ( 'NONE', *, *, #23402, .F. ) ;
#4804=ORIENTED_EDGE ( 'NONE', *, *, #16069, .F. ) ;
#4809=CARTESIAN_POINT ( 'NONE',  ( 16.82730212879999598, -31.88969284570000084, -145.5552959529999839 ) ) ;
#4813=ORIENTED_EDGE ( 'NONE', *, *, #12596, .F. ) ;
#4818=ADVANCED_FACE ( 'NONE', ( #8309 ), #23079, .F. ) ;
#4830=ORIENTED_EDGE ( 'NONE', *, *, #16022, .F. ) ;
#4834=AXIS2_PLACEMENT_3D ( 'NONE', #14100, #23492, #17781 ) ;
#4843=DIRECTION ( 'NONE',  ( 1.000000000000000000, 0.000000000000000000, -8.955190032050000935E-12 ) ) ;
#4846=PLANE ( 'NONE',  #19359 ) ;
#4852=VERTEX_POINT ( 'NONE', #10213 ) ;
#4864=EDGE_LOOP ( 'NONE', ( #4925, #11199, #15718 ) ) ;
#4868=LINE ( 'NONE', #14026, #7583 ) ;
#4870=AXIS2_PLACEMENT_3D ( 'NONE', #7510, #10956, #13214 ) ;
#4874=ORIENTED_EDGE ( 'NONE', *, *, #21808, .F. ) ;
#4875=DIRECTION ( 'NONE',  ( -1.527666881879999979E-13, -8.171241461240000022E-13, -1.000000000000000000 ) ) ;
#4879=ORIENTED_EDGE ( 'NONE', *, *, #11258, .F. ) ;
#4884=DIRECTION ( 'NONE',  ( 2.839308199620000013E-14, 3.568879590630000244E-13, 1.000000000000000000 ) ) ;
#4888=VECTOR ( 'NONE', #18677, 1000.000000000000000 ) ;
#4889=VERTEX_POINT ( 'NONE', #960 ) ;
#4893=DIRECTION ( 'NONE',  ( 0.1720749717299729364, 0.9850838563818457017, -6.484322019408987829E-13 ) ) ;
#4895=CARTESIAN_POINT ( 'NONE',  ( 1.172620240290000115, -63.19354141059999108, -145.5552959529999839 ) ) ;
#4921=( NAMED_UNIT ( * ) PLANE_ANGLE_UNIT ( ) SI_UNIT ( $, .RADIAN. ) );
#4924=EDGE_CURVE ( 'NONE', #1380, #12665, #21659, .T. ) ;
#4925=ORIENTED_EDGE ( 'NONE', *, *, #18827, .F. ) ;
#4928=DIRECTION ( 'NONE',  ( -4.510170015240000199E-12, 1.314504061159999897E-13, -1.000000000000000000 ) ) ;
#4930=EDGE_LOOP ( 'NONE', ( #12417, #18754, #11793 ) ) ;
#4933=CARTESIAN_POINT ( 'NONE',  ( 2.218297500549999857, -15.44723318490000175, -147.5552959529999839 ) ) ;
#4934=EDGE_LOOP ( 'NONE', ( #13852, #23056, #12106, #20693, #9620 ) ) ;
#4947=VERTEX_POINT ( 'NONE', #122 ) ;
#4948=DIRECTION ( 'NONE',  ( 1.000000000000000000, 0.000000000000000000, -8.955799065309598247E-12 ) ) ;
#4951=ORIENTED_EDGE ( 'NONE', *, *, #6206, .F. ) ;
#4962=FACE_OUTER_BOUND ( 'NONE', #14163, .T. ) ;
#4965=DIRECTION ( 'NONE',  ( 1.527666881879999979E-13, 8.100187187669999987E-13, 1.000000000000000000 ) ) ;
#4971=PLANE ( 'NONE',  #60 ) ;
#4986=CARTESIAN_POINT ( 'NONE',  ( -6.601136089949999786, -20.10368962670000315, -144.5552959529999839 ) ) ;
#4996=ORIENTED_EDGE ( 'NONE', *, *, #9777, .T. ) ;
#5009=VECTOR ( 'NONE', #1574, 1000.000000000000000 ) ;
#5013=VECTOR ( 'NONE', #23099, 1000.000000000000114 ) ;
#5016=PLANE ( 'NONE',  #22887 ) ;
#5017=LINE ( 'NONE', #16620, #22507 ) ;
#5025=AXIS2_PLACEMENT_3D ( 'NONE', #4590, #17084, #1161 ) ;
#5044=ORIENTED_EDGE ( 'NONE', *, *, #1826, .F. ) ;
#5049=AXIS2_PLACEMENT_3D ( 'NONE', #12374, #6563, #17743 ) ;
#5051=CARTESIAN_POINT ( 'NONE',  ( -9.347107914279998653, -17.32706600430000066, -144.5552959529999839 ) ) ;
#5052=DIRECTION ( 'NONE',  ( 0.000000000000000000, -1.000000000000000000, 8.159623473500000156E-13 ) ) ;
#5053=ORIENTED_EDGE ( 'NONE', *, *, #19842, .T. ) ;
#5064=DIRECTION ( 'NONE',  ( 0.000000000000000000, -1.000000000000000000, 3.568879590630000244E-13 ) ) ;
#5066=DIRECTION ( 'NONE',  ( 8.955190032050000935E-12, -9.104778821549999739E-13, 1.000000000000000000 ) ) ;
#5078=ORIENTED_EDGE ( 'NONE', *, *, #19723, .T. ) ;
#5116=LINE ( 'NONE', #12252, #16706 ) ;
#5121=DIRECTION ( 'NONE',  ( 9.087266560786239640E-12, 0.000000000000000000, 1.000000000000000000 ) ) ;
#5122=PLANE ( 'NONE',  #17434 ) ;
#5130=LINE ( 'NONE', #19656, #6815 ) ;
#5142=EDGE_CURVE ( 'NONE', #7247, #6997, #6156, .T. ) ;
#5148=CARTESIAN_POINT ( 'NONE',  ( 23.89222110089999873, -31.59487100459999809, -145.5552959529999839 ) ) ;
#5149=EDGE_CURVE ( 'NONE', #23117, #22098, #14967, .T. ) ;
#5152=DIRECTION ( 'NONE',  ( 8.956391184260000029E-12, -9.112710586119999183E-13, 1.000000000000000000 ) ) ;
#5154=AXIS2_PLACEMENT_3D ( 'NONE', #1090, #13815, #21079 ) ;
#5181=LINE ( 'NONE', #7090, #10225 ) ;
#5192=DIRECTION ( 'NONE',  ( -4.430233957459999899E-12, 6.110667527539999876E-13, -1.000000000000000000 ) ) ;
#5193=LINE ( 'NONE', #5440, #21662 ) ;
#5207=ADVANCED_FACE ( 'NONE', ( #8044 ), #10180, .T. ) ;
#5214=DIRECTION ( 'NONE',  ( 2.839308199620000013E-14, 3.568879590630000244E-13, 1.000000000000000000 ) ) ;
#5215=DIRECTION ( 'NONE',  ( -0.09503188512734457583, -0.9954742291034677226, 2.970706163671393545E-13 ) ) ;
#5216=PLANE ( 'NONE',  #10958 ) ;
#5219=VECTOR ( 'NONE', #3601, 1000.000000000000000 ) ;
#5220=VECTOR ( 'NONE', #642, 1000.000000000000114 ) ;
#5226=VERTEX_POINT ( 'NONE', #8277 ) ;
#5229=CARTESIAN_POINT ( 'NONE',  ( -4.946601369560000627, -23.77962690289999870, -144.5552959529999839 ) ) ;
#5231=CARTESIAN_POINT ( 'NONE',  ( 12.82492181439999968, -17.92284828160000032, -145.5552959529999839 ) ) ;
#5235=AXIS2_PLACEMENT_3D ( 'NONE', #7193, #17339, #12663 ) ;
#5244=VERTEX_POINT ( 'NONE', #15786 ) ;
#5246=DIRECTION ( 'NONE',  ( 1.526468026909999897E-13, 8.159623473500000156E-13, 1.000000000000000000 ) ) ;
#5267=CARTESIAN_POINT ( 'NONE',  ( -9.282104535860000283, -16.71402168319999859, -145.5552959529999839 ) ) ;
#5274=CIRCLE ( 'NONE', #18944, 6.000000000000001776 ) ;
#5275=ORIENTED_EDGE ( 'NONE', *, *, #3849, .T. ) ;
#5276=CARTESIAN_POINT ( 'NONE',  ( -9.157754307290000284, -15.75963164970000108, -147.5552959529999839 ) ) ;
#5279=ADVANCED_FACE ( 'NONE', ( #8157 ), #10055, .T. ) ;
#5284=FACE_OUTER_BOUND ( 'NONE', #4930, .T. ) ;
#5287=CARTESIAN_POINT ( 'NONE',  ( -6.165211177139999776, -15.11551140080000089, -142.5552959529999839 ) ) ;
#5293=CIRCLE ( 'NONE', #17453, 15.00000000000000000 ) ;
#5297=ORIENTED_EDGE ( 'NONE', *, *, #9701, .T. ) ;
#5301=LINE ( 'NONE', #80, #15337 ) ;
#5309=VECTOR ( 'NONE', #15433, 1000.000000000000000 ) ;
#5312=AXIS2_PLACEMENT_3D ( 'NONE', #8547, #7255, #6894 ) ;
#5316=VECTOR ( 'NONE', #9696, 1000.000000000000114 ) ;
#5319=AXIS2_PLACEMENT_3D ( 'NONE', #13547, #21299, #23076 ) ;
#5322=ADVANCED_FACE ( 'NONE', ( #4724 ), #20922, .T. ) ;
#5323=ADVANCED_FACE ( 'NONE', ( #13884 ), #10416, .T. ) ;
#5324=CYLINDRICAL_SURFACE ( 'NONE', #20564, 35.00000000000002132 ) ;
#5330=CARTESIAN_POINT ( 'NONE',  ( -6.083910486889999802, -15.16899799649999991, -144.5552959529999839 ) ) ;
#5333=EDGE_CURVE ( 'NONE', #16928, #2852, #10767, .T. ) ;
#5334=DIRECTION ( 'NONE',  ( 0.9989565318111731651, 0.04567108003750790235, -1.889135246290330374E-13 ) ) ;
#5343=ORIENTED_EDGE ( 'NONE', *, *, #10084, .F. ) ;
#5344=LINE ( 'NONE', #1670, #17 ) ;
#5350=VECTOR ( 'NONE', #9725, 1000.000000000000000 ) ;
#5351=CIRCLE ( 'NONE', #20175, 5.999999999999998224 ) ;
#5352=CARTESIAN_POINT ( 'NONE',  ( 7.200097415480000151, -13.39991276200000136, -144.5552959529999839 ) ) ;
#5361=DIRECTION ( 'NONE',  ( -0.9980143568310856361, 0.06298685227120542907, 4.509810669690391193E-12 ) ) ;
#5364=VERTEX_POINT ( 'NONE', #18048 ) ;
#5370=CARTESIAN_POINT ( 'NONE',  ( 5.276897646250000129, -21.39828525539999760, -145.5552959529999839 ) ) ;
#5372=ORIENTED_EDGE ( 'NONE', *, *, #2567, .F. ) ;
#5374=CARTESIAN_POINT ( 'NONE',  ( -6.083910486889999802, -15.16899799649999991, -145.5552959529999839 ) ) ;
#5375=ORIENTED_EDGE ( 'NONE', *, *, #13273, .F. ) ;
#5381=DIRECTION ( 'NONE',  ( -8.955190032050000935E-12, 9.104778821549999739E-13, -1.000000000000000000 ) ) ;
#5392=CYLINDRICAL_SURFACE ( 'NONE', #11041, 14.99999999999999645 ) ;
#5400=DIRECTION ( 'NONE',  ( -0.09606172499277226828, -0.9953753789357124848, 8.265980492677616040E-13 ) ) ;
#5405=AXIS2_PLACEMENT_3D ( 'NONE', #3368, #5621, #3725 ) ;
#5416=FACE_OUTER_BOUND ( 'NONE', #21070, .T. ) ;
#5420=PRODUCT_DEFINITION_CONTEXT ( 'detailed design', #14356, 'design' ) ;
#5438=VECTOR ( 'NONE', #13829, 1000.000000000000114 ) ;
#5440=CARTESIAN_POINT ( 'NONE',  ( -7.041959465309999722, -26.08051538799999847, -143.0552959529999839 ) ) ;
#5459=CYLINDRICAL_SURFACE ( 'NONE', #1157, 4.999999999999999112 ) ;
#5464=ADVANCED_FACE ( 'NONE', ( #19808 ), #15994, .T. ) ;
#5467=DIRECTION ( 'NONE',  ( 0.000000000000000000, -1.000000000000000000, 8.159623473500000156E-13 ) ) ;
#5468=ADVANCED_FACE ( 'NONE', ( #16234 ), #10389, .F. ) ;
#5470=CARTESIAN_POINT ( 'NONE',  ( -9.934356875269999776, -23.16624500709999879, -145.5552959529999839 ) ) ;
#5476=CARTESIAN_POINT ( 'NONE',  ( -6.603585321229999749, -20.59801339440000234, -143.5552959529999839 ) ) ;
#5482=CARTESIAN_POINT ( 'NONE',  ( 2.139623390130000136, -12.81320239329999922, -143.5552959529999839 ) ) ;
#5489=AXIS2_PLACEMENT_3D ( 'NONE', #2680, #9906, #13604 ) ;
#5491=EDGE_CURVE ( 'NONE', #22206, #11516, #21646, .T. ) ;
#5493=ORIENTED_EDGE ( 'NONE', *, *, #23043, .T. ) ;
#5495=VERTEX_POINT ( 'NONE', #14569 ) ;
#5507=ORIENTED_EDGE ( 'NONE', *, *, #17299, .T. ) ;
#5509=DIRECTION ( 'NONE',  ( 4.510774274160000731E-12, -1.321907670990000086E-13, 1.000000000000000000 ) ) ;
#5514=CARTESIAN_POINT ( 'NONE',  ( 4.352290413739999586, -26.01556969399999986, -146.5552959529999839 ) ) ;
#5516=FACE_OUTER_BOUND ( 'NONE', #12806, .T. ) ;
#5519=VECTOR ( 'NONE', #20102, 1000.000000000000000 ) ;
#5521=CARTESIAN_POINT ( 'NONE',  ( -6.477935707790000386, -19.20465386649999928, -146.5552959529999839 ) ) ;
#5522=FACE_OUTER_BOUND ( 'NONE', #11754, .T. ) ;
#5527=EDGE_LOOP ( 'NONE', ( #10291, #1279, #20177, #9571 ) ) ;
#5538=ORIENTED_EDGE ( 'NONE', *, *, #17213, .T. ) ;
#5539=ADVANCED_FACE ( 'NONE', ( #7413 ), #3734, .T. ) ;
#5554=ORIENTED_EDGE ( 'NONE', *, *, #12858, .T. ) ;
#5556=CARTESIAN_POINT ( 'NONE',  ( 24.36715301250000110, -30.57462384669999977, -147.0552959529999839 ) ) ;
#5559=VERTEX_POINT ( 'NONE', #3855 ) ;
#5564=ORIENTED_EDGE ( 'NONE', *, *, #4657, .T. ) ;
#5567=PLANE ( 'NONE',  #8446 ) ;
#5571=LINE ( 'NONE', #12345, #16296 ) ;
#5600=FACE_OUTER_BOUND ( 'NONE', #11412, .T. ) ;
#5608=CARTESIAN_POINT ( 'NONE',  ( 22.40528270640000130, -21.39206583629999869, -146.0552959529999839 ) ) ;
#5609=EDGE_LOOP ( 'NONE', ( #10898, #7639, #10998, #20544, #12176, #3238, #9616 ) ) ;
#5613=EDGE_CURVE ( 'NONE', #919, #15451, #2661, .T. ) ;
#5615=DIRECTION ( 'NONE',  ( -0.9847555042252370550, 0.1739442350240419932, 0.000000000000000000 ) ) ;
#5619=CARTESIAN_POINT ( 'NONE',  ( -9.282104535860000283, -16.71402168319999859, -145.5552959529999839 ) ) ;
#5621=DIRECTION ( 'NONE',  ( 1.526468026909999897E-13, 8.159623473500000156E-13, 1.000000000000000000 ) ) ;
#5624=EDGE_LOOP ( 'NONE', ( #22105, #2816, #2837, #17127, #19060, #2996 ) ) ;
#5626=ORIENTED_EDGE ( 'NONE', *, *, #10962, .T. ) ;
#5627=SURFACE_STYLE_USAGE ( .BOTH. , #22402 ) ;
#5633=CARTESIAN_POINT ( 'NONE',  ( 8.995627988029999855, -17.23072307649999857, -146.5552959529999839 ) ) ;
#5635=DIRECTION ( 'NONE',  ( 9.092994329339670690E-12, 0.000000000000000000, 1.000000000000000000 ) ) ;
#5636=DIRECTION ( 'NONE',  ( 8.740345284041279692E-14, 0.000000000000000000, 1.000000000000000000 ) ) ;
#5641=AXIS2_PLACEMENT_3D ( 'NONE', #11664, #8104, #9438 ) ;
#5646=LINE ( 'NONE', #16834, #16014 ) ;
#5647=LINE ( 'NONE', #13025, #9999 ) ;
#5662=ADVANCED_FACE ( 'NONE', ( #8107 ), #17040, .T. ) ;
#5667=ADVANCED_FACE ( 'NONE', ( #22753 ), #10123, .F. ) ;
#5677=EDGE_LOOP ( 'NONE', ( #13252, #18868, #4237 ) ) ;
#5704=DIRECTION ( 'NONE',  ( 1.000000000000000000, 0.000000000000000000, -8.955534726494208689E-12 ) ) ;
#5710=CARTESIAN_POINT ( 'NONE',  ( -6.599319970649999867, -19.98386714700000155, -145.5552959529999839 ) ) ;
#5718=VECTOR ( 'NONE', #6968, 1000.000000000000000 ) ;
#5722=LINE ( 'NONE', #11180, #259 ) ;
#5727=DIRECTION ( 'NONE',  ( 4.511946372079999833E-12, -1.350031197940000176E-13, 1.000000000000000000 ) ) ;
#5728=EDGE_CURVE ( 'NONE', #22607, #10073, #22287, .T. ) ;
#5742=VERTEX_POINT ( 'NONE', #11669 ) ;
#5745=EDGE_CURVE ( 'NONE', #6134, #21292, #22407, .T. ) ;
#5750=VECTOR ( 'NONE', #12725, 1000.000000000000000 ) ;
#5754=EDGE_CURVE ( 'NONE', #12827, #20361, #5130, .T. ) ;
#5758=DIRECTION ( 'NONE',  ( 0.1146332952500066227, 0.9934078757590583120, 9.947598300640582187E-14 ) ) ;
#5767=LINE ( 'NONE', #14343, #9255 ) ;
#5768=AXIS2_PLACEMENT_3D ( 'NONE', #9290, #2073, #23364 ) ;
#5773=VERTEX_POINT ( 'NONE', #21449 ) ;
#5801=EDGE_CURVE ( 'NONE', #10478, #9593, #6922, .T. ) ;
#5819=DIRECTION ( 'NONE',  ( 0.9996028016287901163, -0.02818224575639410520, -1.295785648389728035E-13 ) ) ;
#5824=DIRECTION ( 'NONE',  ( -2.842170943040000002E-14, -3.552713678800000097E-13, -1.000000000000000000 ) ) ;
#5828=EDGE_CURVE ( 'NONE', #404, #19705, #18587, .T. ) ;
#5829=DIRECTION ( 'NONE',  ( 1.000000000000000000, 0.000000000000000000, -8.954760363766765626E-12 ) ) ;
#5841=LINE ( 'NONE', #14894, #10134 ) ;
#5842=DIRECTION ( 'NONE',  ( 5.228780262857720083E-12, 0.000000000000000000, 1.000000000000000000 ) ) ;
#5854=CARTESIAN_POINT ( 'NONE',  ( 1.342750202250000191, -63.28208324180000233, -144.5552959529999839 ) ) ;
#5859=DIRECTION ( 'NONE',  ( 1.000000000000000000, 0.000000000000000000, -4.510281037539696830E-12 ) ) ;
#5863=VECTOR ( 'NONE', #21326, 1000.000000000000000 ) ;
#5875=EDGE_LOOP ( 'NONE', ( #17390, #14552, #23199, #22850, #17101, #7094, #18541, #6755 ) ) ;
#5879=ADVANCED_FACE ( 'NONE', ( #8465 ), #10362, .T. ) ;
#5884=VECTOR ( 'NONE', #15466, 1000.000000000000000 ) ;
#5894=VERTEX_POINT ( 'NONE', #6681 ) ;
#5911=CARTESIAN_POINT ( 'NONE',  ( 16.82730212879999598, -31.88969284570000084, -146.0552959529999839 ) ) ;
#5916=ORIENTED_EDGE ( 'NONE', *, *, #470, .T. ) ;
#5921=LINE ( 'NONE', #20448, #12498 ) ;
#5945=DIRECTION ( 'NONE',  ( 1.000000000000000000, 0.000000000000000000, -2.715621035259064790E-14 ) ) ;
#5947=FACE_BOUND ( 'NONE', #17091, .T. ) ;
#5953=DIRECTION ( 'NONE',  ( 4.430318231639999944E-12, -6.100259101500000139E-13, 1.000000000000000000 ) ) ;
#5957=EDGE_CURVE ( 'NONE', #7225, #14794, #5921, .T. ) ;
#5959=DIRECTION ( 'NONE',  ( 1.000000000000000000, 0.000000000000000000, -4.511206223393553012E-12 ) ) ;
#5969=FACE_OUTER_BOUND ( 'NONE', #16544, .T. ) ;
#5970=DIRECTION ( 'NONE',  ( 0.4437127003902655575, 0.8961690909155359819, -7.993605777301127091E-13 ) ) ;
#5975=CARTESIAN_POINT ( 'NONE',  ( 2.016283561950000358, -13.16498300129999954, -143.0552959529999839 ) ) ;
#5977=VERTEX_POINT ( 'NONE', #19897 ) ;
#5980=LINE ( 'NONE', #998, #1383 ) ;
#5994=CARTESIAN_POINT ( 'NONE',  ( -9.373415772411227920, -17.59966358942910958, -143.5552959529999839 ) ) ;
#5996=AXIS2_PLACEMENT_3D ( 'NONE', #9870, #17144, #866 ) ;
#5999=EDGE_CURVE ( 'NONE', #14365, #3115, #15174, .T. ) ;
#6010=VECTOR ( 'NONE', #6795, 1000.000000000000000 ) ;
#6018=VERTEX_POINT ( 'NONE', #14544 ) ;
#6024=ORIENTED_EDGE ( 'NONE', *, *, #16214, .T. ) ;
#6032=VECTOR ( 'NONE', #10884, 1000.000000000000000 ) ;
#6035=CIRCLE ( 'NONE', #13643, 5.000000000000000000 ) ;
#6037=VECTOR ( 'NONE', #6910, 1000.000000000000227 ) ;
#6038=ADVANCED_FACE ( 'NONE', ( #15790 ), #4846, .F. ) ;
#6039=CARTESIAN_POINT ( 'NONE',  ( -8.770737564319999180, -11.35481373070000011, -144.5552959529999839 ) ) ;
#6046=EDGE_CURVE ( 'NONE', #11453, #1427, #21160, .T. ) ;
#6060=EDGE_LOOP ( 'NONE', ( #10876, #10070, #19071, #1430 ) ) ;
#6066=AXIS2_PLACEMENT_3D ( 'NONE', #8056, #6280, #13534 ) ;
#6068=CARTESIAN_POINT ( 'NONE',  ( 6.477506801250000557, -13.91317765220000169, -146.5552959529999839 ) ) ;
#6073=ORIENTED_EDGE ( 'NONE', *, *, #22277, .T. ) ;
#6075=EDGE_LOOP ( 'NONE', ( #23400, #16518, #2161 ) ) ;
#6076=AXIS2_PLACEMENT_3D ( 'NONE', #6705, #4695, #5052 ) ;
#6077=AXIS2_PLACEMENT_3D ( 'NONE', #9005, #14510, #16172 ) ;
#6082=CARTESIAN_POINT ( 'NONE',  ( -9.873006318519999880, -23.84776512999999909, -143.0552959529999839 ) ) ;
#6086=LINE ( 'NONE', #17019, #12348 ) ;
#6092=DIRECTION ( 'NONE',  ( 1.000000000000000000, 0.000000000000000000, -8.953948693601887499E-12 ) ) ;
#6094=FACE_OUTER_BOUND ( 'NONE', #7687, .T. ) ;
#6095=AXIS2_PLACEMENT_3D ( 'NONE', #5229, #3457, #10804 ) ;
#6096=AXIS2_PLACEMENT_3D ( 'NONE', #8715, #6948, #23484 ) ;
#6097=ORIENTED_EDGE ( 'NONE', *, *, #3585, .T. ) ;
#6109=CARTESIAN_POINT ( 'NONE',  ( 1.591914056710000080, -18.48847405160000079, -143.5552959529999839 ) ) ;
#6117=DIRECTION ( 'NONE',  ( -0.9954742291034677226, 0.09503188512734457583, 4.503697062742119365E-12 ) ) ;
#6120=CARTESIAN_POINT ( 'NONE',  ( -9.347107914279998653, -17.32706600430000066, -144.5552959529999839 ) ) ;
#6134=VERTEX_POINT ( 'NONE', #14002 ) ;
#6147=ORIENTED_EDGE ( 'NONE', *, *, #5999, .T. ) ;
#6149=LINE ( 'NONE', #5911, #10990 ) ;
#6156=LINE ( 'NONE', #7812, #20854 ) ;
#6158=AXIS2_PLACEMENT_3D ( 'NONE', #19172, #12022, #11780 ) ;
#6162=EDGE_CURVE ( 'NONE', #12155, #21927, #22582, .T. ) ;
#6163=CARTESIAN_POINT ( 'NONE',  ( 16.26251912989999937, -22.62374141290000296, -143.5552959529999839 ) ) ;
#6167=CARTESIAN_POINT ( 'NONE',  ( -9.394779979509999990, -17.86685386420000299, -143.5552959529999839 ) ) ;
#6177=CIRCLE ( 'NONE', #17974, 35.00000000000000000 ) ;
#6189=DIRECTION ( 'NONE',  ( 1.526468026909999897E-13, 8.159623473500000156E-13, 1.000000000000000000 ) ) ;
#6193=ORIENTED_EDGE ( 'NONE', *, *, #17787, .T. ) ;
#6197=CARTESIAN_POINT ( 'NONE',  ( -8.296392858609999976, -9.821782169089999570, -148.5552959529999839 ) ) ;
#6201=EDGE_CURVE ( 'NONE', #22505, #12665, #19718, .T. ) ;
#6202=CARTESIAN_POINT ( 'NONE',  ( 12.77456842470000176, -18.14116071520000162, -143.5552959529999839 ) ) ;
#6206=EDGE_CURVE ( 'NONE', #11246, #1657, #5193, .T. ) ;
#6208=EDGE_CURVE ( 'NONE', #14014, #8887, #12517, .T. ) ;
#6217=EDGE_LOOP ( 'NONE', ( #21375, #4397, #21632, #13982, #224, #22296, #17476 ) ) ;
#6251=CARTESIAN_POINT ( 'NONE',  ( -9.347107914279998653, -17.32706600430000066, -144.5552959529999839 ) ) ;
#6257=EDGE_LOOP ( 'NONE', ( #4225, #18147, #7179, #21923 ) ) ;
#6259=EDGE_CURVE ( 'NONE', #11025, #14032, #3406, .T. ) ;
#6262=DIRECTION ( 'NONE',  ( 0.9915498581664488054, 0.1297261684090585954, -4.315191440381949291E-12 ) ) ;
#6263=DIRECTION ( 'NONE',  ( -0.07970438983373200059, -0.9968185442904001770, 8.265980492683321082E-13 ) ) ;
#6274=LINE ( 'NONE', #22350, #10148 ) ;
#6278=DIRECTION ( 'NONE',  ( -0.9847555042252370550, 0.1739442350240419932, 0.000000000000000000 ) ) ;
#6279=VERTEX_POINT ( 'NONE', #19602 ) ;
#6280=DIRECTION ( 'NONE',  ( -0.9953753789357124848, 0.09606172499277225441, 7.355811845627876534E-14 ) ) ;
#6290=FACE_BOUND ( 'NONE', #18411, .T. ) ;
#6292=CARTESIAN_POINT ( 'NONE',  ( 24.11847952820000174, -31.58456057200000089, -143.5552959529999839 ) ) ;
#6293=ORIENTED_EDGE ( 'NONE', *, *, #7650, .T. ) ;
#6295=LINE ( 'NONE', #8185, #18616 ) ;
#6298=EDGE_CURVE ( 'NONE', #7247, #21766, #16386, .T. ) ;
#6302=CARTESIAN_POINT ( 'NONE',  ( 23.89222110089999873, -31.59487100459999809, -146.5552959529999839 ) ) ;
#6306=DIRECTION ( 'NONE',  ( 1.000000000000000000, 0.000000000000000000, -4.510774274160000731E-12 ) ) ;
#6318=DIRECTION ( 'NONE',  ( 1.000000000000000000, 0.000000000000000000, -8.955190032050000935E-12 ) ) ;
#6324=AXIS2_PLACEMENT_3D ( 'NONE', #14799, #13006, #16118 ) ;
#6325=DIRECTION ( 'NONE',  ( 1.526468026909860048E-13, 8.159623473498529972E-13, 1.000000000000000000 ) ) ;
#6326=ORIENTED_EDGE ( 'NONE', *, *, #19836, .F. ) ;
#6347=ORIENTED_EDGE ( 'NONE', *, *, #819, .T. ) ;
#6352=DIRECTION ( 'NONE',  ( 1.526468026909999897E-13, 8.159623473500000156E-13, 1.000000000000000000 ) ) ;
#6369=ORIENTED_EDGE ( 'NONE', *, *, #854, .T. ) ;
#6376=CARTESIAN_POINT ( 'NONE',  ( -9.347107914279998653, -17.32706600430000066, -143.5552959529999839 ) ) ;
#6379=LINE ( 'NONE', #11602, #3749 ) ;
#6393=VERTEX_POINT ( 'NONE', #9682 ) ;
#6408=ORIENTED_EDGE ( 'NONE', *, *, #21475, .T. ) ;
#6421=CARTESIAN_POINT ( 'NONE',  ( 5.347956485829999274, -22.34165470570000167, -147.5552959529999839 ) ) ;
#6424=DIRECTION ( 'NONE',  ( 4.510774274160000731E-12, -1.321907670990000086E-13, 1.000000000000000000 ) ) ;
#6429=VECTOR ( 'NONE', #19170, 999.9999999999998863 ) ;
#6435=ORIENTED_EDGE ( 'NONE', *, *, #22602, .F. ) ;
#6443=ORIENTED_EDGE ( 'NONE', *, *, #8853, .F. ) ;
#6446=VECTOR ( 'NONE', #13559, 1000.000000000000000 ) ;
#6460=CARTESIAN_POINT ( 'NONE',  ( 1.561837858109999866, -18.84848306830000197, -143.5552959529999839 ) ) ;
#6467=AXIS2_PLACEMENT_3D ( 'NONE', #13254, #655, #4101 ) ;
#6479=ORIENTED_EDGE ( 'NONE', *, *, #3308, .T. ) ;
#6492=ORIENTED_EDGE ( 'NONE', *, *, #13323, .T. ) ;
#6493=DIRECTION ( 'NONE',  ( -0.9874789572432817186, 0.1577507813030449846, 0.000000000000000000 ) ) ;
#6500=ORIENTED_EDGE ( 'NONE', *, *, #3308, .F. ) ;
#6516=DIRECTION ( 'NONE',  ( 1.000000000000000000, 0.000000000000000000, -1.498801083243961330E-13 ) ) ;
#6517=FACE_OUTER_BOUND ( 'NONE', #3350, .T. ) ;
#6522=CARTESIAN_POINT ( 'NONE',  ( 15.97954986339999905, -26.72957102550000030, -143.0552959529999839 ) ) ;
#6528=ADVANCED_FACE ( 'NONE', ( #8722 ), #21601, .F. ) ;
#6529=EDGE_LOOP ( 'NONE', ( #17919, #7385, #12798, #21642 ) ) ;
#6530=DIRECTION ( 'NONE',  ( -0.09606172499277226828, -0.9953753789357124848, 8.268133652477615271E-13 ) ) ;
#6531=DIRECTION ( 'NONE',  ( 1.527666881879999979E-13, 8.100187187669999987E-13, 1.000000000000000000 ) ) ;
#6535=AXIS2_PLACEMENT_3D ( 'NONE', #20495, #7632, #6092 ) ;
#6537=CARTESIAN_POINT ( 'NONE',  ( 23.84377886109999878, -30.60602870049999780, -145.0552959529999839 ) ) ;
#6541=LINE ( 'NONE', #15591, #12011 ) ;
#6542=LINE ( 'NONE', #6421, #5884 ) ;
#6544=CARTESIAN_POINT ( 'NONE',  ( -7.337311498550000088, -24.10744501490000147, -148.0552959529999839 ) ) ;
#6545=VERTEX_POINT ( 'NONE', #16001 ) ;
#6548=VECTOR ( 'NONE', #6531, 1000.000000000000000 ) ;
#6550=PLANE ( 'NONE',  #694 ) ;
#6556=DIRECTION ( 'NONE',  ( 4.510774274160000731E-12, -1.321907670990000086E-13, 1.000000000000000000 ) ) ;
#6557=DIRECTION ( 'NONE',  ( 4.510774274160000731E-12, -1.321907670990000086E-13, 1.000000000000000000 ) ) ;
#6559=ADVANCED_FACE ( 'NONE', ( #5284 ), #7188, .T. ) ;
#6563=DIRECTION ( 'NONE',  ( 2.839308199620000013E-14, 3.568879590630000244E-13, 1.000000000000000000 ) ) ;
#6586=EDGE_CURVE ( 'NONE', #23020, #6018, #21724, .T. ) ;
#6588=VERTEX_POINT ( 'NONE', #21484 ) ;
#6589=DIRECTION ( 'NONE',  ( 1.000000000000000000, 0.000000000000000000, -4.429789868254373788E-12 ) ) ;
#6593=EDGE_CURVE ( 'NONE', #4852, #2114, #7856, .T. ) ;
#6605=EDGE_CURVE ( 'NONE', #21627, #4564, #15875, .T. ) ;
#6608=ADVANCED_FACE ( 'NONE', ( #19686 ), #3383, .T. ) ;
#6610=DIRECTION ( 'NONE',  ( 0.9896415801065049367, -0.1435602414469282218, -8.993136838065500309E-12 ) ) ;
#6612=ORIENTED_EDGE ( 'NONE', *, *, #11852, .T. ) ;
#6630=DIRECTION ( 'NONE',  ( 1.000000000000000000, 0.000000000000000000, -2.775557561562891351E-14 ) ) ;
#6632=CARTESIAN_POINT ( 'NONE',  ( 23.78818517497548513, -17.51387386322154072, -148.5552959529998418 ) ) ;
#6633=PLANE ( 'NONE',  #15809 ) ;
#6643=ORIENTED_EDGE ( 'NONE', *, *, #12079, .T. ) ;
#6647=DIRECTION ( 'NONE',  ( -0.1435602414469281940, -0.9896415801065048257, 3.849849731938073961E-13 ) ) ;
#6651=ORIENTED_EDGE ( 'NONE', *, *, #2842, .T. ) ;
#6657=FACE_OUTER_BOUND ( 'NONE', #13549, .T. ) ;
#6661=PLANE ( 'NONE',  #10645 ) ;
#6662=CARTESIAN_POINT ( 'NONE',  ( -9.056357402059999728, -12.43025388040000045, -147.5552959529999839 ) ) ;
#6665=VECTOR ( 'NONE', #9772, 999.9999999999998863 ) ;
#6671=CARTESIAN_POINT ( 'NONE',  ( 22.01137100460000084, -15.39610142400000115, -147.5552959529999839 ) ) ;
#6681=CARTESIAN_POINT ( 'NONE',  ( 1.693247834384973283, -17.47463886119383503, -146.5552959530003250 ) ) ;
#6694=CARTESIAN_POINT ( 'NONE',  ( -2.491922975426976272, -28.49278486398841181, -144.5552959529864552 ) ) ;
#6698=VECTOR ( 'NONE', #19460, 1000.000000000000000 ) ;
#6701=LINE ( 'NONE', #21116, #17253 ) ;
#6705=CARTESIAN_POINT ( 'NONE',  ( -9.347107914279998653, -17.32706600430000066, -144.5552959529999839 ) ) ;
#6710=DIRECTION ( 'NONE',  ( 1.000000000000000000, 0.000000000000000000, -4.510281037539699253E-12 ) ) ;
#6711=ADVANCED_FACE ( 'NONE', ( #5522 ), #13122, .F. ) ;
#6714=DIRECTION ( 'NONE',  ( -4.510774274160000731E-12, 1.321907670990000086E-13, -1.000000000000000000 ) ) ;
#6715=CARTESIAN_POINT ( 'NONE',  ( 23.93638409349999918, -31.59322175579999836, -144.5552959529999839 ) ) ;
#6718=EDGE_LOOP ( 'NONE', ( #17930, #7128, #7658, #14718, #588 ) ) ;
#6726=DIRECTION ( 'NONE',  ( -0.1146332952500066227, -0.9934078757590583120, -9.947598300640582187E-14 ) ) ;
#6732=DIRECTION ( 'NONE',  ( 4.430318231639999944E-12, -6.100259101500000139E-13, 1.000000000000000000 ) ) ;
#6733=DIRECTION ( 'NONE',  ( -0.9748402797454081004, 0.2229045288590935092, 4.454830202381862158E-12 ) ) ;
#6734=CARTESIAN_POINT ( 'NONE',  ( 16.87269471589999981, -31.91616505980000085, -144.0552959529999839 ) ) ;
#6737=DIRECTION ( 'NONE',  ( 1.000000000000000000, 0.000000000000000000, -8.955190032050000935E-12 ) ) ;
#6743=CARTESIAN_POINT ( 'NONE',  ( 1.393351898023278412, -20.95564341188169522, -143.5552959529982218 ) ) ;
#6744=VECTOR ( 'NONE', #21311, 1000.000000000000000 ) ;
#6747=PLANE ( 'NONE',  #21906 ) ;
#6750=LINE ( 'NONE', #10541, #11087 ) ;
#6755=ORIENTED_EDGE ( 'NONE', *, *, #16548, .F. ) ;
#6757=LINE ( 'NONE', #17712, #8322 ) ;
#6759=ORIENTED_EDGE ( 'NONE', *, *, #5728, .T. ) ;
#6765=VECTOR ( 'NONE', #12448, 1000.000000000000000 ) ;
#6772=CARTESIAN_POINT ( 'NONE',  ( -8.770737564319999180, -11.35481373070000011, -144.5552959529999839 ) ) ;
#6783=CARTESIAN_POINT ( 'NONE',  ( -4.021770264099999714, -29.17051924670000318, -143.0552959529999839 ) ) ;
#6784=AXIS2_PLACEMENT_3D ( 'NONE', #243, #9719, #4385 ) ;
#6785=ORIENTED_EDGE ( 'NONE', *, *, #15697, .T. ) ;
#6788=FACE_OUTER_BOUND ( 'NONE', #13904, .T. ) ;
#6789=CARTESIAN_POINT ( 'NONE',  ( 21.44117969379999877, -21.36894679869999791, -147.5552959529999839 ) ) ;
#6790=CARTESIAN_POINT ( 'NONE',  ( 7.200097415480000151, -13.39991276200000136, -144.5552959529999839 ) ) ;
#6791=CARTESIAN_POINT ( 'NONE',  ( 12.81474735470000148, -17.96536370379999781, -144.5552959529999839 ) ) ;
#6792=VERTEX_POINT ( 'NONE', #9658 ) ;
#6794=ADVANCED_FACE ( 'NONE', ( #10010 ), #20744, .T. ) ;
#6795=DIRECTION ( 'NONE',  ( -4.510170015240000199E-12, 1.314504061159999897E-13, -1.000000000000000000 ) ) ;
#6801=ORIENTED_EDGE ( 'NONE', *, *, #21508, .T. ) ;
#6805=CIRCLE ( 'NONE', #17837, 9.999999999999998224 ) ;
#6808=ORIENTED_EDGE ( 'NONE', *, *, #16973, .F. ) ;
#6811=CARTESIAN_POINT ( 'NONE',  ( -6.477935707790000386, -19.20465386649999928, -146.5552959529999839 ) ) ;
#6815=VECTOR ( 'NONE', #8572, 999.9999999999998863 ) ;
#6817=VERTEX_POINT ( 'NONE', #8354 ) ;
#6822=ORIENTED_EDGE ( 'NONE', *, *, #8631, .F. ) ;
#6825=CARTESIAN_POINT ( 'NONE',  ( 5.792747474879999636, -16.92794981449999980, -145.5552959529999839 ) ) ;
#6826=VECTOR ( 'NONE', #22603, 1000.000000000000000 ) ;
#6827=LINE ( 'NONE', #3154, #6836 ) ;
#6831=CARTESIAN_POINT ( 'NONE',  ( 7.558347240409999834, -12.62842008530000015, -147.5552959529999839 ) ) ;
#6835=FACE_OUTER_BOUND ( 'NONE', #2247, .T. ) ;
#6836=VECTOR ( 'NONE', #10383, 1000.000000000000000 ) ;
#6839=AXIS2_PLACEMENT_3D ( 'NONE', #325, #21984, #9238 ) ;
#6843=UNCERTAINTY_MEASURE_WITH_UNIT (LENGTH_MEASURE( 1.000000000000000082E-05 ), #16105, 'distance_accuracy_value', 'NONE');
#6845=ORIENTED_EDGE ( 'NONE', *, *, #470, .F. ) ;
#6853=DIRECTION ( 'NONE',  ( 1.000000000000000000, 0.000000000000000000, -4.430318231639999944E-12 ) ) ;
#6854=EDGE_CURVE ( 'NONE', #9593, #20938, #1596, .T. ) ;
#6857=STYLED_ITEM ( 'NONE', ( #13113 ), #11538 ) ;
#6859=ORIENTED_EDGE ( 'NONE', *, *, #17213, .F. ) ;
#6862=CARTESIAN_POINT ( 'NONE',  ( 1.172620240290000115, -63.19354141059999108, -145.5552959529999839 ) ) ;
#6866=DIRECTION ( 'NONE',  ( 0.04459224566432164888, 0.9990052710704848682, -8.219575497233998330E-13 ) ) ;
#6867=DIRECTION ( 'NONE',  ( 8.645353842254780479E-13, 0.000000000000000000, -1.000000000000000000 ) ) ;
#6869=EDGE_CURVE ( 'NONE', #20874, #9011, #12506, .T. ) ;
#6878=ORIENTED_EDGE ( 'NONE', *, *, #19836, .T. ) ;
#6880=DIRECTION ( 'NONE',  ( 1.000000000000000000, 0.000000000000000000, -8.954760363766765626E-12 ) ) ;
#6894=DIRECTION ( 'NONE',  ( 1.000000000000000000, 0.000000000000000000, -8.953948693601887499E-12 ) ) ;
#6895=EDGE_LOOP ( 'NONE', ( #9583, #207, #23122, #6435, #8029, #12422 ) ) ;
#6910=DIRECTION ( 'NONE',  ( -0.1146332952500066227, -0.9934078757590583120, -1.023181539490060155E-13 ) ) ;
#6911=EDGE_CURVE ( 'NONE', #14227, #2700, #21554, .T. ) ;
#6914=LINE ( 'NONE', #10816, #19169 ) ;
#6915=ORIENTED_EDGE ( 'NONE', *, *, #15793, .F. ) ;
#6921=CIRCLE ( 'NONE', #6158, 2.999999999999999112 ) ;
#6922=LINE ( 'NONE', #14298, #18976 ) ;
#6924=EDGE_CURVE ( 'NONE', #16352, #11025, #1052, .T. ) ;
#6928=CARTESIAN_POINT ( 'NONE',  ( 22.42591623494620023, -15.34961090601114542, -144.5552959529997281 ) ) ;
#6936=VERTEX_POINT ( 'NONE', #12385 ) ;
#6942=DIRECTION ( 'NONE',  ( 0.1435602414469281940, 0.9896415801065048257, -3.836930773098079160E-13 ) ) ;
#6948=DIRECTION ( 'NONE',  ( 0.9953753789357124848, -0.09606172499277225441, -7.355811845627870223E-14 ) ) ;
#6953=CARTESIAN_POINT ( 'NONE',  ( -2.100773033209999863, -15.22510554480000167, -145.5552959529999839 ) ) ;
#6960=EDGE_CURVE ( 'NONE', #14794, #23501, #1470, .T. ) ;
#6965=LINE ( 'NONE', #18035, #9493 ) ;
#6968=DIRECTION ( 'NONE',  ( 1.527666881879999979E-13, 8.171241461240000022E-13, 1.000000000000000000 ) ) ;
#6978=DIRECTION ( 'NONE',  ( 1.000000000000000000, 0.000000000000000000, -2.775557561562892298E-14 ) ) ;
#6979=AXIS2_PLACEMENT_3D ( 'NONE', #8298, #9317, #1867 ) ;
#6997=VERTEX_POINT ( 'NONE', #12274 ) ;
#7020=FACE_OUTER_BOUND ( 'NONE', #20341, .T. ) ;
#7030=ORIENTED_EDGE ( 'NONE', *, *, #574, .T. ) ;
#7032=PLANE ( 'NONE',  #20835 ) ;
#7035=CARTESIAN_POINT ( 'NONE',  ( 21.39890631740000160, -21.26106171180000359, -145.5552959529999839 ) ) ;
#7039=CARTESIAN_POINT ( 'NONE',  ( 5.631397321050000571, -17.85059010000000157, -147.5552959529999839 ) ) ;
#7045=DIRECTION ( 'NONE',  ( 0.07970438983373200059, 0.9968185442904001770, -8.242295734823311485E-13 ) ) ;
#7047=DIRECTION ( 'NONE',  ( 1.000000000000000000, 0.000000000000000000, -8.955799065309598247E-12 ) ) ;
#7048=ORIENTED_EDGE ( 'NONE', *, *, #9356, .F. ) ;
#7057=ADVANCED_FACE ( 'NONE', ( #15002 ), #152, .T. ) ;
#7065=EDGE_CURVE ( 'NONE', #11626, #19736, #20365, .T. ) ;
#7079=CIRCLE ( 'NONE', #4042, 5.000000000000000000 ) ;
#7081=UNCERTAINTY_MEASURE_WITH_UNIT (LENGTH_MEASURE( 1.000000000000000082E-05 ), #23244, 'distance_accuracy_value', 'NONE');
#7086=CYLINDRICAL_SURFACE ( 'NONE', #12217, 6.000000000000002665 ) ;
#7090=CARTESIAN_POINT ( 'NONE',  ( -6.477935707790000386, -19.20465386649999928, -147.5552959529999839 ) ) ;
#7093=FACE_OUTER_BOUND ( 'NONE', #9335, .T. ) ;
#7094=ORIENTED_EDGE ( 'NONE', *, *, #19127, .F. ) ;
#7095=CARTESIAN_POINT ( 'NONE',  ( -6.083910486889999802, -15.16899799649999991, -144.5552959529999839 ) ) ;
#7097=CARTESIAN_POINT ( 'NONE',  ( -9.157754307290000284, -15.75963164970000108, -147.5552959529999839 ) ) ;
#7102=VERTEX_POINT ( 'NONE', #11182 ) ;
#7110=EDGE_LOOP ( 'NONE', ( #23352, #1144, #10089, #21539, #13397, #1941 ) ) ;
#7114=ORIENTED_EDGE ( 'NONE', *, *, #6593, .F. ) ;
#7115=ORIENTED_EDGE ( 'NONE', *, *, #20640, .F. ) ;
#7117=EDGE_CURVE ( 'NONE', #22329, #14876, #7736, .T. ) ;
#7118=DIRECTION ( 'NONE',  ( 1.000000000000000000, 0.000000000000000000, -4.430318231639999944E-12 ) ) ;
#7123=CARTESIAN_POINT ( 'NONE',  ( -6.657076963140000636, -20.13603737529999904, -144.5552959529999839 ) ) ;
#7128=ORIENTED_EDGE ( 'NONE', *, *, #959, .T. ) ;
#7130=LINE ( 'NONE', #8782, #579 ) ;
#7136=DIRECTION ( 'NONE',  ( 4.430318231639999944E-12, -6.100259101500000139E-13, 1.000000000000000000 ) ) ;
#7142=VECTOR ( 'NONE', #8696, 1000.000000000000114 ) ;
#7150=CARTESIAN_POINT ( 'NONE',  ( -7.149448239889999890, -25.45628515800000002, -146.5552959529999839 ) ) ;
#7168=EDGE_CURVE ( 'NONE', #361, #1717, #966, .T. ) ;
#7172=PLANE ( 'NONE',  #20680 ) ;
#7177=CIRCLE ( 'NONE', #1489, 8.176568160360000448 ) ;
#7179=ORIENTED_EDGE ( 'NONE', *, *, #23218, .T. ) ;
#7182=CIRCLE ( 'NONE', #20863, 8.176568160360000448 ) ;
#7188=PLANE ( 'NONE',  #3700 ) ;
#7192=AXIS2_PLACEMENT_3D ( 'NONE', #13468, #15380, #11443 ) ;
#7193=CARTESIAN_POINT ( 'NONE',  ( 2.508811538190000245, -14.35090895149999923, -145.5552959529999839 ) ) ;
#7195=EDGE_LOOP ( 'NONE', ( #2436, #19501, #10737 ) ) ;
#7199=ADVANCED_FACE ( 'NONE', ( #20957 ), #11529, .F. ) ;
#7210=EDGE_CURVE ( 'NONE', #320, #19030, #13568, .T. ) ;
#7211=CARTESIAN_POINT ( 'NONE',  ( -4.160432423080000497, -28.71743394529999804, -143.5552959529999839 ) ) ;
#7216=VECTOR ( 'NONE', #12564, 1000.000000000000227 ) ;
#7217=ORIENTED_EDGE ( 'NONE', *, *, #1689, .T. ) ;
#7220=VECTOR ( 'NONE', #9058, 1000.000000000000114 ) ;
#7222=VECTOR ( 'NONE', #9716, 999.9999999999998863 ) ;
#7225=VERTEX_POINT ( 'NONE', #17258 ) ;
#7227=EDGE_LOOP ( 'NONE', ( #2090, #6193, #13763, #10007 ) ) ;
#7229=DIRECTION ( 'NONE',  ( 0.9944529286486341046, -0.1051825684329612265, -4.469111776238355154E-12 ) ) ;
#7246=CARTESIAN_POINT ( 'NONE',  ( 17.66940543669999997, -18.68690163239999791, -144.5552959529999839 ) ) ;
#7247=VERTEX_POINT ( 'NONE', #15117 ) ;
#7250=VERTEX_POINT ( 'NONE', #20711 ) ;
#7255=DIRECTION ( 'NONE',  ( 8.955190032050000935E-12, -9.104778821549999739E-13, 1.000000000000000000 ) ) ;
#7264=ORIENTED_EDGE ( 'NONE', *, *, #3283, .F. ) ;
#7274=CARTESIAN_POINT ( 'NONE',  ( -9.812199629320000227, -24.40642616239999896, -147.0552959529999839 ) ) ;
#7289=DIRECTION ( 'NONE',  ( -0.9847555042252370550, 0.1739442350240419932, 7.083477032991710236E-15 ) ) ;
#7295=ORIENTED_EDGE ( 'NONE', *, *, #3963, .T. ) ;
#7302=AXIS2_PLACEMENT_3D ( 'NONE', #13075, #20576, #5704 ) ;
#7305=AXIS2_PLACEMENT_3D ( 'NONE', #720, #18795, #18907 ) ;
#7307=DIRECTION ( 'NONE',  ( 8.955190032050000935E-12, -9.104778821549999739E-13, 1.000000000000000000 ) ) ;
#7308=CARTESIAN_POINT ( 'NONE',  ( -6.165211177139999776, -15.11551140080000089, -143.5552959529999839 ) ) ;
#7313=DIRECTION ( 'NONE',  ( -0.9938526945756316344, 0.1107105301439589573, 6.178155812097707047E-14 ) ) ;
#7315=ORIENTED_EDGE ( 'NONE', *, *, #11192, .F. ) ;
#7319=ORIENTED_EDGE ( 'NONE', *, *, #23058, .T. ) ;
#7329=DIRECTION ( 'NONE',  ( -0.09606172499277214338, -0.9953753789357123738, 8.234154099303244678E-13 ) ) ;
#7331=LINE ( 'NONE', #14354, #15609 ) ;
#7337=DIRECTION ( 'NONE',  ( -2.839308199620000013E-14, -3.568879590630000244E-13, -1.000000000000000000 ) ) ;
#7340=EDGE_CURVE ( 'NONE', #8156, #16928, #6274, .T. ) ;
#7347=ORIENTED_EDGE ( 'NONE', *, *, #13135, .T. ) ;
#7356=CARTESIAN_POINT ( 'NONE',  ( 6.841811532420000397, -13.03968765259999962, -144.5552959529999839 ) ) ;
#7357=CARTESIAN_POINT ( 'NONE',  ( 5.631397321050000571, -17.85059010000000157, -146.5552959529999839 ) ) ;
#7368=EDGE_CURVE ( 'NONE', #13630, #15489, #16986, .T. ) ;
#7372=VERTEX_POINT ( 'NONE', #11615 ) ;
#7375=CARTESIAN_POINT ( 'NONE',  ( 23.84377886109999878, -30.60602870049999780, -144.5552959529999839 ) ) ;
#7376=CARTESIAN_POINT ( 'NONE',  ( -8.857008087982999101, -12.44928454996512635, -146.5552959529661621 ) ) ;
#7385=ORIENTED_EDGE ( 'NONE', *, *, #9407, .T. ) ;
#7386=VECTOR ( 'NONE', #6942, 1000.000000000000000 ) ;
#7411=SURFACE_STYLE_FILL_AREA ( #11200 ) ;
#7413=FACE_OUTER_BOUND ( 'NONE', #13734, .T. ) ;
#7426=ORIENTED_EDGE ( 'NONE', *, *, #7168, .T. ) ;
#7428=FACE_OUTER_BOUND ( 'NONE', #14560, .T. ) ;
#7433=DIRECTION ( 'NONE',  ( -0.9892101392001054760, 0.1465035852930155480, 4.471489433380478225E-12 ) ) ;
#7438=EDGE_CURVE ( 'NONE', #4564, #10851, #18154, .T. ) ;
#7451=VERTEX_POINT ( 'NONE', #3630 ) ;
#7464=DIRECTION ( 'NONE',  ( -2.839308199620000013E-14, -3.568879590630000244E-13, -1.000000000000000000 ) ) ;
#7465=LINE ( 'NONE', #22112, #15536 ) ;
#7467=DIRECTION ( 'NONE',  ( -4.430233957459999899E-12, 6.110667527539999876E-13, -1.000000000000000000 ) ) ;
#7470=VERTEX_POINT ( 'NONE', #2951 ) ;
#7473=EDGE_CURVE ( 'NONE', #22736, #18669, #2832, .T. ) ;
#7489=CARTESIAN_POINT ( 'NONE',  ( 2.048233066679999936, -63.64014441970000746, -143.0552959529999839 ) ) ;
#7490=EDGE_CURVE ( 'NONE', #5244, #20874, #12415, .T. ) ;
#7493=EDGE_CURVE ( 'NONE', #2813, #9406, #8259, .T. ) ;
#7499=CARTESIAN_POINT ( 'NONE',  ( -9.434278515689999978, -18.41834002140000237, -147.5552959529999839 ) ) ;
#7507=CARTESIAN_POINT ( 'NONE',  ( -9.394779979509999990, -17.86685386420000299, -143.5552959529999839 ) ) ;
#7510=CARTESIAN_POINT ( 'NONE',  ( 24.59017985859999911, -26.91621017459999976, -148.5552959529999839 ) ) ;
#7512=VECTOR ( 'NONE', #9484, 1000.000000000000114 ) ;
#7517=CARTESIAN_POINT ( 'NONE',  ( -9.969904307360000217, -22.67446893780000039, -145.5552959529999839 ) ) ;
#7523=CARTESIAN_POINT ( 'NONE',  ( -6.320468577110000652, -16.70961797440000041, -146.5552959529999839 ) ) ;
#7524=VECTOR ( 'NONE', #13502, 1000.000000000000000 ) ;
#7530=LINE ( 'NONE', #4089, #5220 ) ;
#7544=AXIS2_PLACEMENT_3D ( 'NONE', #19735, #1544, #18063 ) ;
#7546=AXIS2_PLACEMENT_3D ( 'NONE', #22495, #6189, #22257 ) ;
#7547=CARTESIAN_POINT ( 'NONE',  ( 6.841811532410000396, -13.03968765259999962, -145.5552959529999839 ) ) ;
#7557=ORIENTED_EDGE ( 'NONE', *, *, #6924, .F. ) ;
#7565=EDGE_LOOP ( 'NONE', ( #15686, #6651, #324, #13795, #7114, #1051 ) ) ;
#7568=EDGE_LOOP ( 'NONE', ( #14582, #3544, #17746, #10892 ) ) ;
#7576=LINE ( 'NONE', #7804, #17852 ) ;
#7578=DIRECTION ( 'NONE',  ( 2.839308199620000013E-14, 3.568879590630000244E-13, 1.000000000000000000 ) ) ;
#7579=VECTOR ( 'NONE', #2711, 1000.000000000000114 ) ;
#7581=AXIS2_PLACEMENT_3D ( 'NONE', #18785, #7940, #15224 ) ;
#7583=VECTOR ( 'NONE', #19393, 999.9999999999998863 ) ;
#7586=FACE_OUTER_BOUND ( 'NONE', #3059, .T. ) ;
#7587=ORIENTED_EDGE ( 'NONE', *, *, #12709, .T. ) ;
#7603=EDGE_LOOP ( 'NONE', ( #15226, #7587, #6759, #345, #2229, #20910, #4353, #7264 ) ) ;
#7606=DIRECTION ( 'NONE',  ( 0.7739965043580748771, 0.6331898698190620012, -3.042011087472929325E-12 ) ) ;
#7608=DIRECTION ( 'NONE',  ( 1.000000000000000000, 0.000000000000000000, -2.854859206178974232E-14 ) ) ;
#7616=ORIENTED_EDGE ( 'NONE', *, *, #5999, .F. ) ;
#7617=DIRECTION ( 'NONE',  ( 1.526468026909860048E-13, 8.159623473498529972E-13, 1.000000000000000000 ) ) ;
#7632=DIRECTION ( 'NONE',  ( 8.955190032050000935E-12, -9.104778821549999739E-13, 1.000000000000000000 ) ) ;
#7635=ORIENTED_EDGE ( 'NONE', *, *, #20641, .T. ) ;
#7639=ORIENTED_EDGE ( 'NONE', *, *, #5491, .T. ) ;
#7641=DIRECTION ( 'NONE',  ( 1.526468026909655070E-13, 8.159623473495709763E-13, 1.000000000000000000 ) ) ;
#7643=VECTOR ( 'NONE', #2763, 1000.000000000000000 ) ;
#7650=EDGE_CURVE ( 'NONE', #1168, #7247, #20397, .T. ) ;
#7657=DIRECTION ( 'NONE',  ( -4.430318231639999944E-12, 6.100259101500000139E-13, -1.000000000000000000 ) ) ;
#7658=ORIENTED_EDGE ( 'NONE', *, *, #10463, .T. ) ;
#7661=LINE ( 'NONE', #16942, #21754 ) ;
#7664=CIRCLE ( 'NONE', #6535, 5.000000000000000000 ) ;
#7665=ORIENTED_EDGE ( 'NONE', *, *, #2567, .T. ) ;
#7673=EDGE_CURVE ( 'NONE', #22550, #2114, #2327, .T. ) ;
#7687=EDGE_LOOP ( 'NONE', ( #22713, #13671, #18155, #18114, #5078, #7790, #976, #10524 ) ) ;
#7689=VERTEX_POINT ( 'NONE', #20993 ) ;
#7691=LINE ( 'NONE', #17093, #14420 ) ;
#7701=CARTESIAN_POINT ( 'NONE',  ( 8.327852746066881195, -18.10800434007730786, -146.5552959530281782 ) ) ;
#7703=EDGE_CURVE ( 'NONE', #9187, #1380, #19441, .T. ) ;
#7710=LINE ( 'NONE', #18670, #2953 ) ;
#7713=ORIENTED_EDGE ( 'NONE', *, *, #4003, .F. ) ;
#7728=ORIENTED_EDGE ( 'NONE', *, *, #23341, .T. ) ;
#7732=EDGE_CURVE ( 'NONE', #10602, #19256, #17756, .T. ) ;
#7736=LINE ( 'NONE', #37, #7872 ) ;
#7738=ORIENTED_EDGE ( 'NONE', *, *, #1252, .T. ) ;
#7741=PLANE ( 'NONE',  #4870 ) ;
#7746=AXIS2_PLACEMENT_3D ( 'NONE', #21939, #11084, #1839 ) ;
#7749=LINE ( 'NONE', #15133, #18316 ) ;
#7751=EDGE_CURVE ( 'NONE', #20549, #18609, #4066, .T. ) ;
#7755=ORIENTED_EDGE ( 'NONE', *, *, #10283, .T. ) ;
#7763=VECTOR ( 'NONE', #2050, 1000.000000000000114 ) ;
#7766=CARTESIAN_POINT ( 'NONE',  ( 12.82492181439999968, -17.92284828160000032, -146.5552959529999839 ) ) ;
#7769=VERTEX_POINT ( 'NONE', #3955 ) ;
#7770=EDGE_CURVE ( 'NONE', #20679, #17230, #21595, .T. ) ;
#7772=ORIENTED_EDGE ( 'NONE', *, *, #14244, .T. ) ;
#7773=ORIENTED_EDGE ( 'NONE', *, *, #10084, .T. ) ;
#7774=DIRECTION ( 'NONE',  ( 2.842170943040000002E-14, 3.552713678800000097E-13, 1.000000000000000000 ) ) ;
#7778=DIRECTION ( 'NONE',  ( 1.000000000000000000, 0.000000000000000000, -8.955799065309598247E-12 ) ) ;
#7790=ORIENTED_EDGE ( 'NONE', *, *, #12513, .F. ) ;
#7791=VECTOR ( 'NONE', #20867, 1000.000000000000114 ) ;
#7804=CARTESIAN_POINT ( 'NONE',  ( -9.157754307299999397, -15.75963164970000108, -148.5552959529999839 ) ) ;
#7805=EDGE_CURVE ( 'NONE', #4889, #8373, #9286, .T. ) ;
#7807=DIRECTION ( 'NONE',  ( 1.000000000000000000, 0.000000000000000000, -8.955534726494208689E-12 ) ) ;
#7812=CARTESIAN_POINT ( 'NONE',  ( 17.66940543669999997, -18.68690163239999791, -145.0552959529999839 ) ) ;
#7830=ORIENTED_EDGE ( 'NONE', *, *, #16868, .F. ) ;
#7832=PLANE ( 'NONE',  #2324 ) ;
#7841=EDGE_LOOP ( 'NONE', ( #7830, #19843, #15165 ) ) ;
#7845=ADVANCED_FACE ( 'NONE', ( #16559 ), #7741, .F. ) ;
#7849=ORIENTED_EDGE ( 'NONE', *, *, #3555, .T. ) ;
#7856=CIRCLE ( 'NONE', #10895, 9.999999999999998224 ) ;
#7863=CARTESIAN_POINT ( 'NONE',  ( 24.85988213910000155, -26.16224997189999968, -144.5552959529999839 ) ) ;
#7866=CARTESIAN_POINT ( 'NONE',  ( 9.438695624090803094, -28.66738265459707691, -147.5552959529370582 ) ) ;
#7872=VECTOR ( 'NONE', #9041, 999.9999999999998863 ) ;
#7873=DIRECTION ( 'NONE',  ( 0.1720749717299729364, 0.9850838563818457017, -6.484322019408987829E-13 ) ) ;
#7885=DIRECTION ( 'NONE',  ( 1.526468026909999897E-13, 8.159623473500000156E-13, 1.000000000000000000 ) ) ;
#7889=DIRECTION ( 'NONE',  ( -0.9874789572432817186, 0.1577507813030449846, 2.556342494820729215E-14 ) ) ;
#7897=ORIENTED_EDGE ( 'NONE', *, *, #10482, .F. ) ;
#7898=VECTOR ( 'NONE', #852, 1000.000000000000000 ) ;
#7899=ADVANCED_FACE ( 'NONE', ( #17021 ), #6550, .F. ) ;
#7901=EDGE_CURVE ( 'NONE', #21292, #5364, #22618, .T. ) ;
#7902=FACE_OUTER_BOUND ( 'NONE', #10253, .T. ) ;
#7903=VECTOR ( 'NONE', #2043, 1000.000000000000114 ) ;
#7905=DIRECTION ( 'NONE',  ( -0.9954742291034677226, 0.09503188512734457583, 4.503363594322118746E-12 ) ) ;
#7906=EDGE_CURVE ( 'NONE', #1168, #11590, #10104, .T. ) ;
#7909=AXIS2_PLACEMENT_3D ( 'NONE', #19624, #3442, #3676 ) ;
#7918=CARTESIAN_POINT ( 'NONE',  ( 24.89581725840000104, -26.85672394480000236, -144.5552959529999839 ) ) ;
#7923=VERTEX_POINT ( 'NONE', #1093 ) ;
#7940=DIRECTION ( 'NONE',  ( 8.955190032049920155E-12, -9.104778821555109033E-13, 1.000000000000000000 ) ) ;
#7945=AXIS2_PLACEMENT_3D ( 'NONE', #16419, #4034, #129 ) ;
#7950=DIRECTION ( 'NONE',  ( 4.533528609800090131E-12, 0.000000000000000000, 1.000000000000000000 ) ) ;
#7954=DIRECTION ( 'NONE',  ( 8.955190032050000935E-12, -9.104778821549999739E-13, 1.000000000000000000 ) ) ;
#7955=FACE_OUTER_BOUND ( 'NONE', #2927, .T. ) ;
#7961=VECTOR ( 'NONE', #19805, 1000.000000000000227 ) ;
#7968=ADVANCED_FACE ( 'NONE', ( #8092 ), #18928, .F. ) ;
#7972=DIRECTION ( 'NONE',  ( -0.9832226533249337486, 0.1824094679249879947, 1.246536736419916629E-15 ) ) ;
#7973=PLANE ( 'NONE',  #18829 ) ;
#7985=CARTESIAN_POINT ( 'NONE',  ( -7.337311498550000088, -24.10744501490000147, -148.5552959529999839 ) ) ;
#7986=ORIENTED_EDGE ( 'NONE', *, *, #7901, .F. ) ;
#8024=VECTOR ( 'NONE', #10488, 1000.000000000000114 ) ;
#8025=CIRCLE ( 'NONE', #17566, 35.00000000000000000 ) ;
#8029=ORIENTED_EDGE ( 'NONE', *, *, #2127, .F. ) ;
#8034=ORIENTED_EDGE ( 'NONE', *, *, #13135, .F. ) ;
#8044=FACE_OUTER_BOUND ( 'NONE', #9451, .T. ) ;
#8051=CARTESIAN_POINT ( 'NONE',  ( -8.823001505574659120, -11.89636386765829812, -143.5552959529989892 ) ) ;
#8055=ORIENTED_EDGE ( 'NONE', *, *, #15697, .F. ) ;
#8056=CARTESIAN_POINT ( 'NONE',  ( 15.87827223000000032, -26.60524292859999917, -143.5552959529999839 ) ) ;
#8057=LINE ( 'NONE', #6522, #16032 ) ;
#8071=CARTESIAN_POINT ( 'NONE',  ( 22.40884248670000289, -21.39641658300000060, -143.5552959529999839 ) ) ;
#8073=LINE ( 'NONE', #10083, #6826 ) ;
#8080=ADVANCED_FACE ( 'NONE', ( #3458 ), #10451, .T. ) ;
#8090=CARTESIAN_POINT ( 'NONE',  ( 22.27792782919999937, -15.32580087659999890, -145.5552959529999839 ) ) ;
#8092=FACE_OUTER_BOUND ( 'NONE', #833, .T. ) ;
#8093=DIRECTION ( 'NONE',  ( -0.9840552701943220404, 0.1778629393740580045, 0.000000000000000000 ) ) ;
#8098=DIRECTION ( 'NONE',  ( -0.9913873220698726785, 0.1309625047069831461, -1.853446743629759619E-14 ) ) ;
#8102=DIRECTION ( 'NONE',  ( 1.000000000000000000, 0.000000000000000000, -1.526556658859589738E-13 ) ) ;
#8103=EDGE_CURVE ( 'NONE', #12665, #19198, #13926, .T. ) ;
#8104=DIRECTION ( 'NONE',  ( 1.526468026910264955E-13, 8.159623473499449847E-13, 1.000000000000000000 ) ) ;
#8107=FACE_OUTER_BOUND ( 'NONE', #17292, .T. ) ;
#8108=ORIENTED_EDGE ( 'NONE', *, *, #21890, .F. ) ;
#8116=AXIS2_PLACEMENT_3D ( 'NONE', #14668, #17893, #20033 ) ;
#8137=EDGE_CURVE ( 'NONE', #19198, #17357, #5116, .T. ) ;
#8146=ORIENTED_EDGE ( 'NONE', *, *, #8806, .F. ) ;
#8156=VERTEX_POINT ( 'NONE', #356 ) ;
#8157=FACE_OUTER_BOUND ( 'NONE', #18300, .T. ) ;
#8160=VECTOR ( 'NONE', #7313, 999.9999999999998863 ) ;
#8161=CARTESIAN_POINT ( 'NONE',  ( 1.713198289059999935, -17.44292009260000142, -148.5552959529999839 ) ) ;
#8162=ORIENTED_EDGE ( 'NONE', *, *, #19273, .T. ) ;
#8170=CARTESIAN_POINT ( 'NONE',  ( -6.072796602490000417, -14.62912504250000012, -143.5552959529999839 ) ) ;
#8185=CARTESIAN_POINT ( 'NONE',  ( 16.16922456049999823, -22.27514461170000004, -147.5552959529999839 ) ) ;
#8189=ORIENTED_EDGE ( 'NONE', *, *, #23203, .T. ) ;
#8191=ADVANCED_FACE ( 'NONE', ( #478 ), #14980, .T. ) ;
#8196=CARTESIAN_POINT ( 'NONE',  ( 1.364575185789999923, -21.31553777220000256, -142.5552959529999839 ) ) ;
#8203=EDGE_CURVE ( 'NONE', #13434, #7451, #2150, .T. ) ;
#8209=CARTESIAN_POINT ( 'NONE',  ( -7.337311498540000088, -24.10744501490000147, -147.5552959529999839 ) ) ;
#8211=CARTESIAN_POINT ( 'NONE',  ( -9.895958504584086768, -22.78427602437751176, -145.5552959529979660 ) ) ;
#8219=AXIS2_PLACEMENT_3D ( 'NONE', #1153, #21372, #10155 ) ;
#8241=VERTEX_POINT ( 'NONE', #16306 ) ;
#8245=DIRECTION ( 'NONE',  ( 0.9944529286486341046, -0.1051825684329612265, -4.470295960598355531E-12 ) ) ;
#8249=DIRECTION ( 'NONE',  ( -0.9846904924346530086, 0.1743118874569384857, 8.976860394976840322E-12 ) ) ;
#8251=CARTESIAN_POINT ( 'NONE',  ( 23.40529971389999986, -31.60139774330000151, -148.0552959529999839 ) ) ;
#8256=ORIENTED_EDGE ( 'NONE', *, *, #23341, .F. ) ;
#8257=CARTESIAN_POINT ( 'NONE',  ( 6.477506801250000557, -13.91317765220000169, -147.5552959529999839 ) ) ;
#8259=CIRCLE ( 'NONE', #5235, 15.00000000000000000 ) ;
#8263=CARTESIAN_POINT ( 'NONE',  ( 16.61718498210000305, -18.75502267109999721, -143.5552959529999839 ) ) ;
#8265=EDGE_LOOP ( 'NONE', ( #18182, #3363, #19871, #14432, #6369, #19598, #19837 ) ) ;
#8270=LINE ( 'NONE', #1169, #13665 ) ;
#8276=EDGE_LOOP ( 'NONE', ( #4801, #10669, #21986, #11479 ) ) ;
#8277=CARTESIAN_POINT ( 'NONE',  ( 23.84377886109999878, -30.60602870049999780, -145.5552959529999839 ) ) ;
#8297=AXIS2_PLACEMENT_3D ( 'NONE', #11850, #8407, #15680 ) ;
#8298=CARTESIAN_POINT ( 'NONE',  ( -8.594304764359998572, -10.75357442870000035, -145.5552959529999839 ) ) ;
#8302=CARTESIAN_POINT ( 'NONE',  ( -9.790691201043280500, -24.06562932247060260, -147.5552959529991313 ) ) ;
#8304=DIRECTION ( 'NONE',  ( 0.1435602414469281940, 0.9896415801065048257, -3.836930773098079160E-13 ) ) ;
#8307=VECTOR ( 'NONE', #3346, 1000.000000000000227 ) ;
#8309=FACE_OUTER_BOUND ( 'NONE', #8265, .T. ) ;
#8310=ORIENTED_EDGE ( 'NONE', *, *, #14834, .T. ) ;
#8311=VERTEX_POINT ( 'NONE', #7376 ) ;
#8316=CARTESIAN_POINT ( 'NONE',  ( 2.508811538200000246, -14.35090895149999923, -144.5552959529999839 ) ) ;
#8317=DIRECTION ( 'NONE',  ( 0.9989565318111731651, 0.04567108003750790235, -1.889135246290330374E-13 ) ) ;
#8322=VECTOR ( 'NONE', #1425, 999.9999999999998863 ) ;
#8323=CARTESIAN_POINT ( 'NONE',  ( -7.041959465309999722, -26.08051538799999847, -143.5552959529999839 ) ) ;
#8330=CARTESIAN_POINT ( 'NONE',  ( 2.048233066679999936, -63.64014441970000746, -142.5552959529999839 ) ) ;
#8334=LINE ( 'NONE', #3229, #17269 ) ;
#8343=AXIS2_PLACEMENT_3D ( 'NONE', #11934, #6352, #23016 ) ;
#8345=AXIS2_PLACEMENT_3D ( 'NONE', #955, #22714, #13672 ) ;
#8354=CARTESIAN_POINT ( 'NONE',  ( 1.799591341878497452, -16.33655707908583565, -144.5552959529918553 ) ) ;
#8355=DIRECTION ( 'NONE',  ( 0.1435602414469281940, 0.9896415801065048257, -3.836930773098079160E-13 ) ) ;
#8369=EDGE_CURVE ( 'NONE', #6817, #18344, #19019, .T. ) ;
#8372=CARTESIAN_POINT ( 'NONE',  ( -6.615063969075902328, -20.14048105937242283, -145.5552959529732391 ) ) ;
#8373=VERTEX_POINT ( 'NONE', #8170 ) ;
#8389=ORIENTED_EDGE ( 'NONE', *, *, #6960, .F. ) ;
#8393=DIRECTION ( 'NONE',  ( 2.839308199620000013E-14, 3.568879590630000244E-13, 1.000000000000000000 ) ) ;
#8399=PLANE ( 'NONE',  #14814 ) ;
#8402=LINE ( 'NONE', #15895, #23006 ) ;
#8404=EDGE_CURVE ( 'NONE', #14970, #23117, #589, .T. ) ;
#8406=ORIENTED_EDGE ( 'NONE', *, *, #8369, .F. ) ;
#8407=DIRECTION ( 'NONE',  ( 4.510774274160000731E-12, -1.321907670990000086E-13, 1.000000000000000000 ) ) ;
#8412=ORIENTED_EDGE ( 'NONE', *, *, #7703, .F. ) ;
#8415=FACE_OUTER_BOUND ( 'NONE', #3447, .T. ) ;
#8416=ORIENTED_EDGE ( 'NONE', *, *, #10004, .T. ) ;
#8425=ORIENTED_EDGE ( 'NONE', *, *, #3565, .T. ) ;
#8428=PLANE ( 'NONE',  #19472 ) ;
#8446=AXIS2_PLACEMENT_3D ( 'NONE', #23308, #14506, #7118 ) ;
#8449=DIRECTION ( 'NONE',  ( -0.9847555042252370550, 0.1739442350240419932, 7.303835699471759765E-15 ) ) ;
#8451=ORIENTED_EDGE ( 'NONE', *, *, #4430, .F. ) ;
#8454=CARTESIAN_POINT ( 'NONE',  ( 2.139623390130000136, -12.81320239329999922, -144.5552959529999839 ) ) ;
#8462=ADVANCED_FACE ( 'NONE', ( #19136 ), #11506, .T. ) ;
#8465=FACE_OUTER_BOUND ( 'NONE', #22472, .T. ) ;
#8470=CARTESIAN_POINT ( 'NONE',  ( 2.218297500559999857, -15.44723318490000175, -146.5552959529999839 ) ) ;
#8478=FACE_OUTER_BOUND ( 'NONE', #16128, .T. ) ;
#8480=ADVANCED_FACE ( 'NONE', ( #17116 ), #834, .T. ) ;
#8485=ORIENTED_EDGE ( 'NONE', *, *, #12807, .F. ) ;
#8511=VECTOR ( 'NONE', #6117, 999.9999999999998863 ) ;
#8518=DIRECTION ( 'NONE',  ( 8.955190032050000935E-12, -9.104778821549999739E-13, 1.000000000000000000 ) ) ;
#8523=ORIENTED_EDGE ( 'NONE', *, *, #16973, .T. ) ;
#8524=CARTESIAN_POINT ( 'NONE',  ( 24.85988213910000155, -26.16224997189999968, -145.0552959529999839 ) ) ;
#8535=EDGE_LOOP ( 'NONE', ( #13070, #685, #2328, #19965 ) ) ;
#8547=CARTESIAN_POINT ( 'NONE',  ( -5.070907855429999778, -22.41528233759999722, -147.5552959529999839 ) ) ;
#8556=AXIS2_PLACEMENT_3D ( 'NONE', #16795, #22616, #2760 ) ;
#8563=CARTESIAN_POINT ( 'NONE',  ( 17.06104532839999877, -32.02344838739999489, -143.5552959529999839 ) ) ;
#8565=CARTESIAN_POINT ( 'NONE',  ( 21.44117969379999877, -21.36894679869999791, -147.0552959529999839 ) ) ;
#8572=DIRECTION ( 'NONE',  ( -0.09606172499277226828, -0.9953753789357124848, 8.268133652477615271E-13 ) ) ;
#8580=LINE ( 'NONE', #1250, #975 ) ;
#8591=ORIENTED_EDGE ( 'NONE', *, *, #11131, .T. ) ;
#8596=DIRECTION ( 'NONE',  ( 4.510774274157260696E-12, -1.321907671014926071E-13, 1.000000000000000000 ) ) ;
#8597=LINE ( 'NONE', #6831, #15430 ) ;
#8598=CARTESIAN_POINT ( 'NONE',  ( 12.91075631260000023, -38.04527125359999928, -147.5552959529999839 ) ) ;
#8600=VECTOR ( 'NONE', #21370, 1000.000000000000000 ) ;
#8609=ORIENTED_EDGE ( 'NONE', *, *, #2845, .F. ) ;
#8627=EDGE_CURVE ( 'NONE', #13656, #22550, #757, .T. ) ;
#8629=ORIENTED_EDGE ( 'NONE', *, *, #2136, .F. ) ;
#8631=EDGE_CURVE ( 'NONE', #34, #21613, #21480, .T. ) ;
#8632=LINE ( 'NONE', #21163, #21720 ) ;
#8649=CARTESIAN_POINT ( 'NONE',  ( 24.87050155979999744, -26.86223000240000047, -146.0552959529999839 ) ) ;
#8658=PLANE ( 'NONE',  #19956 ) ;
#8665=CARTESIAN_POINT ( 'NONE',  ( 7.200097415480000151, -13.39991276200000136, -143.5552959529999839 ) ) ;
#8666=VECTOR ( 'NONE', #18524, 1000.000000000000000 ) ;
#8668=DIRECTION ( 'NONE',  ( 0.9834926989016489207, 0.1809478134909354718, -4.411697319228424767E-12 ) ) ;
#8685=ADVANCED_FACE ( 'NONE', ( #12062 ), #21245, .F. ) ;
#8696=DIRECTION ( 'NONE',  ( -0.06298685227120542907, -0.9980143568310855251, 1.534772309240130738E-13 ) ) ;
#8697=DIRECTION ( 'NONE',  ( 8.955190032050000935E-12, -9.104778821549999739E-13, 1.000000000000000000 ) ) ;
#8706=CARTESIAN_POINT ( 'NONE',  ( 22.27731556082403941, -15.33058227694559683, -144.5552959530006945 ) ) ;
#8712=AXIS2_PLACEMENT_3D ( 'NONE', #9504, #9379, #5945 ) ;
#8715=CARTESIAN_POINT ( 'NONE',  ( 1.829659965300000080, -16.02499107890000118, -143.5552959529999839 ) ) ;
#8721=DIRECTION ( 'NONE',  ( 4.430233957459999899E-12, -6.110667527539999876E-13, 1.000000000000000000 ) ) ;
#8722=FACE_OUTER_BOUND ( 'NONE', #20905, .T. ) ;
#8725=VECTOR ( 'NONE', #12401, 1000.000000000000114 ) ;
#8726=DIRECTION ( 'NONE',  ( 4.510774274159160626E-12, -1.321907670996266040E-13, 1.000000000000000000 ) ) ;
#8733=ORIENTED_EDGE ( 'NONE', *, *, #14269, .T. ) ;
#8735=ORIENTED_EDGE ( 'NONE', *, *, #3666, .T. ) ;
#8756=DIRECTION ( 'NONE',  ( 1.526468026909999897E-13, 8.159623473500000156E-13, 1.000000000000000000 ) ) ;
#8758=DIRECTION ( 'NONE',  ( 1.000000000000000000, 0.000000000000000000, -4.429789868254375404E-12 ) ) ;
#8774=EDGE_CURVE ( 'NONE', #18274, #20361, #3737, .T. ) ;
#8782=CARTESIAN_POINT ( 'NONE',  ( 7.228490359739999427, -13.33508289800000135, -145.5552959529999839 ) ) ;
#8788=PLANE ( 'NONE',  #5154 ) ;
#8792=LINE ( 'NONE', #23443, #4614 ) ;
#8795=VERTEX_POINT ( 'NONE', #14452 ) ;
#8805=CARTESIAN_POINT ( 'NONE',  ( -9.282104535860000283, -16.71402168319999859, -145.5552959529999839 ) ) ;
#8806=EDGE_CURVE ( 'NONE', #1178, #5495, #1550, .T. ) ;
#8808=LINE ( 'NONE', #12495, #8307 ) ;
#8810=CARTESIAN_POINT ( 'NONE',  ( -4.192924954330000453, -28.60725908990000121, -145.5552959529999839 ) ) ;
#8819=ORIENTED_EDGE ( 'NONE', *, *, #20012, .F. ) ;
#8824=EDGE_LOOP ( 'NONE', ( #4951, #3313, #7728, #13688 ) ) ;
#8826=SHAPE_REPRESENTATION_RELATIONSHIP ( 'NONE' , 'NONE' ,  #15746, #1875 ) ;
#8830=FACE_OUTER_BOUND ( 'NONE', #9036, .T. ) ;
#8834=ORIENTED_EDGE ( 'NONE', *, *, #19273, .F. ) ;
#8843=CARTESIAN_POINT ( 'NONE',  ( -6.072796602490000417, -14.62912504250000012, -143.5552959529999839 ) ) ;
#8851=ORIENTED_EDGE ( 'NONE', *, *, #10821, .T. ) ;
#8853=EDGE_CURVE ( 'NONE', #7102, #19545, #9863, .T. ) ;
#8858=CARTESIAN_POINT ( 'NONE',  ( 23.19105773460000108, -15.44374190390000123, -146.5552959529999839 ) ) ;
#8867=FACE_OUTER_BOUND ( 'NONE', #10656, .T. ) ;
#8879=DIRECTION ( 'NONE',  ( -0.1000233216789610108, -0.9949850929136109245, 3.591470555298595137E-13 ) ) ;
#8881=EDGE_CURVE ( 'NONE', #4947, #1178, #2843, .T. ) ;
#8883=DIRECTION ( 'NONE',  ( 1.000000000000000000, 0.000000000000000000, -4.429789868254374596E-12 ) ) ;
#8887=VERTEX_POINT ( 'NONE', #21877 ) ;
#8903=EDGE_LOOP ( 'NONE', ( #4830, #2316 ) ) ;
#8919=EDGE_CURVE ( 'NONE', #5495, #10871, #19614, .T. ) ;
#8928=DIRECTION ( 'NONE',  ( -2.842170943040000002E-14, -3.552713678800000097E-13, -1.000000000000000000 ) ) ;
#8931=EDGE_LOOP ( 'NONE', ( #9130, #917, #7347, #22447, #10098 ) ) ;
#8939=EDGE_LOOP ( 'NONE', ( #7986, #10632, #1076, #18039 ) ) ;
#8943=LINE ( 'NONE', #16224, #81 ) ;
#8955=DIRECTION ( 'NONE',  ( 4.511946372079999833E-12, -1.314504061159999897E-13, 1.000000000000000000 ) ) ;
#8967=ORIENTED_EDGE ( 'NONE', *, *, #13614, .T. ) ;
#8971=ORIENTED_EDGE ( 'NONE', *, *, #4591, .F. ) ;
#8980=VERTEX_POINT ( 'NONE', #23416 ) ;
#8983=EDGE_CURVE ( 'NONE', #14014, #8887, #22421, .T. ) ;
#8985=CARTESIAN_POINT ( 'NONE',  ( -4.959431410700000598, -23.66636161550000139, -146.5552959529999839 ) ) ;
#8988=ORIENTED_EDGE ( 'NONE', *, *, #2099, .F. ) ;
#8994=ORIENTED_EDGE ( 'NONE', *, *, #15638, .T. ) ;
#9005=CARTESIAN_POINT ( 'NONE',  ( -4.888913597060000171, -24.24628707910000003, -142.5552959529999839 ) ) ;
#9009=AXIS2_PLACEMENT_3D ( 'NONE', #11893, #4529, #4408 ) ;
#9011=VERTEX_POINT ( 'NONE', #15192 ) ;
#9019=FACE_OUTER_BOUND ( 'NONE', #15448, .T. ) ;
#9023=VERTEX_POINT ( 'NONE', #13049 ) ;
#9024=CARTESIAN_POINT ( 'NONE',  ( 2.068499633500000545, -14.99362786250000035, -148.5552959529999839 ) ) ;
#9032=LINE ( 'NONE', #16319, #12089 ) ;
#9036=EDGE_LOOP ( 'NONE', ( #17260, #2840, #82, #21830, #18319 ) ) ;
#9038=VECTOR ( 'NONE', #20007, 1000.000000000000114 ) ;
#9041=DIRECTION ( 'NONE',  ( -0.9954742291034677226, 0.09503188512734457583, 4.503697062742119365E-12 ) ) ;
#9050=DIRECTION ( 'NONE',  ( -0.1146332952500066227, -0.9934078757590583120, -9.710750722050572275E-14 ) ) ;
#9058=DIRECTION ( 'NONE',  ( -0.9892101392001054760, 0.1465035852930155480, 4.471739159800472250E-12 ) ) ;
#9059=LINE ( 'NONE', #14209, #20155 ) ;
#9065=AXIS2_PLACEMENT_3D ( 'NONE', #13063, #342, #20334 ) ;
#9068=CARTESIAN_POINT ( 'NONE',  ( 1.342750202250000191, -63.28208324180000233, -143.5552959529999839 ) ) ;
#9075=CARTESIAN_POINT ( 'NONE',  ( 1.600095057559999923, -18.40127899619999852, -145.5552959529999839 ) ) ;
#9080=ORIENTED_EDGE ( 'NONE', *, *, #14904, .F. ) ;
#9088=DIRECTION ( 'NONE',  ( -0.09606172499277226828, -0.9953753789357124848, 8.268133652477615271E-13 ) ) ;
#9093=ADVANCED_FACE ( 'NONE', ( #11136 ), #4123, .F. ) ;
#9096=PLANE ( 'NONE',  #1436 ) ;
#9103=VECTOR ( 'NONE', #16288, 1000.000000000000000 ) ;
#9106=VECTOR ( 'NONE', #1554, 1000.000000000000000 ) ;
#9110=ORIENTED_EDGE ( 'NONE', *, *, #8983, .T. ) ;
#9128=CARTESIAN_POINT ( 'NONE',  ( 17.58326321919999558, -18.99156222550000095, -146.5552959529999839 ) ) ;
#9129=DIRECTION ( 'NONE',  ( 0.1051825684329612265, 0.9944529286486342157, 1.406498023189481106E-13 ) ) ;
#9130=ORIENTED_EDGE ( 'NONE', *, *, #21006, .F. ) ;
#9137=CARTESIAN_POINT ( 'NONE',  ( 24.35183050010000017, -28.38413933620000051, -144.5552959529999839 ) ) ;
#9156=PLANE ( 'NONE',  #22213 ) ;
#9161=CARTESIAN_POINT ( 'NONE',  ( -9.394779979509999990, -17.86685386420000299, -143.5552959529999839 ) ) ;
#9170=VECTOR ( 'NONE', #8668, 1000.000000000000114 ) ;
#9171=CIRCLE ( 'NONE', #22491, 5.000000000000000000 ) ;
#9182=FACE_OUTER_BOUND ( 'NONE', #3170, .T. ) ;
#9187=VERTEX_POINT ( 'NONE', #22805 ) ;
#9188=VECTOR ( 'NONE', #9465, 1000.000000000000000 ) ;
#9189=PLANE ( 'NONE',  #6096 ) ;
#9194=DIRECTION ( 'NONE',  ( 1.526468026909860048E-13, 8.159623473498529972E-13, 1.000000000000000000 ) ) ;
#9199=ADVANCED_FACE ( 'NONE', ( #18871 ), #10169, .T. ) ;
#9207=VERTEX_POINT ( 'NONE', #4473 ) ;
#9216=CYLINDRICAL_SURFACE ( 'NONE', #17037, 3.000000000000000000 ) ;
#9217=ORIENTED_EDGE ( 'NONE', *, *, #16572, .T. ) ;
#9225=ORIENTED_EDGE ( 'NONE', *, *, #23137, .F. ) ;
#9238=DIRECTION ( 'NONE',  ( 1.000000000000000000, 0.000000000000000000, -4.510774274160000731E-12 ) ) ;
#9242=ORIENTED_EDGE ( 'NONE', *, *, #21186, .T. ) ;
#9248=PLANE ( 'NONE',  #14005 ) ;
#9249=ORIENTED_EDGE ( 'NONE', *, *, #22913, .T. ) ;
#9253=LINE ( 'NONE', #21894, #18876 ) ;
#9255=VECTOR ( 'NONE', #9088, 999.9999999999998863 ) ;
#9264=LINE ( 'NONE', #13307, #13753 ) ;
#9266=ORIENTED_EDGE ( 'NONE', *, *, #14469, .F. ) ;
#9269=CARTESIAN_POINT ( 'NONE',  ( 23.93638409349999918, -31.59322175579999836, -144.5552959529999839 ) ) ;
#9270=PLANE ( 'NONE',  #17958 ) ;
#9277=ORIENTED_EDGE ( 'NONE', *, *, #737, .T. ) ;
#9279=EDGE_CURVE ( 'NONE', #11485, #1998, #6965, .T. ) ;
#9286=LINE ( 'NONE', #14555, #22342 ) ;
#9290=CARTESIAN_POINT ( 'NONE',  ( 24.87050155979999744, -26.86223000240000047, -146.5552959529999839 ) ) ;
#9292=FACE_OUTER_BOUND ( 'NONE', #2239, .T. ) ;
#9298=CARTESIAN_POINT ( 'NONE',  ( 1.354168148130000082, -20.95195702430000040, -144.5552959529999839 ) ) ;
#9310=ORIENTED_EDGE ( 'NONE', *, *, #23058, .F. ) ;
#9313=AXIS2_PLACEMENT_3D ( 'NONE', #19438, #3246, #10479 ) ;
#9316=VECTOR ( 'NONE', #18632, 1000.000000000000000 ) ;
#9317=DIRECTION ( 'NONE',  ( -0.9934078757590584230, 0.1146332952500066366, 4.471042303700267278E-12 ) ) ;
#9322=ORIENTED_EDGE ( 'NONE', *, *, #18117, .T. ) ;
#9332=CARTESIAN_POINT ( 'NONE',  ( 7.795574410691926026, -18.05719095672263563, -147.5552959530097894 ) ) ;
#9333=ORIENTED_EDGE ( 'NONE', *, *, #20130, .F. ) ;
#9335=EDGE_LOOP ( 'NONE', ( #9369, #6347, #18737, #9394 ) ) ;
#9349=PLANE ( 'NONE',  #2616 ) ;
#9353=ORIENTED_EDGE ( 'NONE', *, *, #7438, .T. ) ;
#9356=EDGE_CURVE ( 'NONE', #15779, #20935, #1388, .T. ) ;
#9359=ORIENTED_EDGE ( 'NONE', *, *, #8103, .T. ) ;
#9369=ORIENTED_EDGE ( 'NONE', *, *, #14244, .F. ) ;
#9371=DIRECTION ( 'NONE',  ( -0.9874789572432817186, 0.1577507813030449846, 2.125043109900604696E-14 ) ) ;
#9377=LINE ( 'NONE', #22139, #15928 ) ;
#9379=DIRECTION ( 'NONE',  ( 2.839308199620000013E-14, 3.568879590630000244E-13, 1.000000000000000000 ) ) ;
#9394=ORIENTED_EDGE ( 'NONE', *, *, #16522, .F. ) ;
#9399=DIRECTION ( 'NONE',  ( 1.526468026909999897E-13, 8.159623473500000156E-13, 1.000000000000000000 ) ) ;
#9405=DIRECTION ( 'NONE',  ( 0.000000000000000000, -7.444689577964079813E-14, -1.000000000000000000 ) ) ;
#9406=VERTEX_POINT ( 'NONE', #8211 ) ;
#9407=EDGE_CURVE ( 'NONE', #21983, #1038, #2877, .T. ) ;
#9409=ADVANCED_FACE ( 'NONE', ( #6788 ), #5122, .F. ) ;
#9411=CARTESIAN_POINT ( 'NONE',  ( -7.129475577410000042, -25.57825421080000083, -143.5552959529999839 ) ) ;
#9416=ORIENTED_EDGE ( 'NONE', *, *, #1826, .T. ) ;
#9426=AXIS2_PLACEMENT_3D ( 'NONE', #18210, #3816, #19994 ) ;
#9433=EDGE_CURVE ( 'NONE', #20938, #8241, #21322, .T. ) ;
#9434=VECTOR ( 'NONE', #16201, 1000.000000000000114 ) ;
#9435=CARTESIAN_POINT ( 'NONE',  ( -8.916553640509999212, -11.88594259849999979, -143.0552959529999839 ) ) ;
#9438=DIRECTION ( 'NONE',  ( 0.4293832457559224602, -0.9031223772358367707, 6.707597440443650396E-13 ) ) ;
#9444=VECTOR ( 'NONE', #13507, 1000.000000000000227 ) ;
#9451=EDGE_LOOP ( 'NONE', ( #17121, #2054, #16150, #22839, #15413, #3348 ) ) ;
#9465=DIRECTION ( 'NONE',  ( -8.955280961229999814E-12, 9.094947017729999296E-13, -1.000000000000000000 ) ) ;
#9470=VECTOR ( 'NONE', #13186, 1000.000000000000000 ) ;
#9472=EDGE_LOOP ( 'NONE', ( #7849, #962, #9266, #10081 ) ) ;
#9484=DIRECTION ( 'NONE',  ( 0.1720749717299729364, 0.9850838563818457017, -6.484322019408987829E-13 ) ) ;
#9486=VECTOR ( 'NONE', #17543, 1000.000000000000227 ) ;
#9489=ORIENTED_EDGE ( 'NONE', *, *, #8203, .T. ) ;
#9493=VECTOR ( 'NONE', #15888, 1000.000000000000000 ) ;
#9496=EDGE_LOOP ( 'NONE', ( #10368, #2550, #9080, #13419, #21816 ) ) ;
#9503=ADVANCED_FACE ( 'NONE', ( #4662 ), #22983, .F. ) ;
#9504=CARTESIAN_POINT ( 'NONE',  ( 2.170391987449999505, -12.72823260819999902, -145.5552959529999839 ) ) ;
#9506=DIRECTION ( 'NONE',  ( -1.526468026909999897E-13, -8.159623473500000156E-13, -1.000000000000000000 ) ) ;
#9510=VECTOR ( 'NONE', #8245, 1000.000000000000114 ) ;
#9511=EDGE_CURVE ( 'NONE', #4754, #20005, #15164, .T. ) ;
#9514=CARTESIAN_POINT ( 'NONE',  ( 2.139623390130000136, -12.81320239329999922, -144.0552959529999839 ) ) ;
#9520=DIRECTION ( 'NONE',  ( 1.526468026909999897E-13, 8.159623473500000156E-13, 1.000000000000000000 ) ) ;
#9526=EDGE_CURVE ( 'NONE', #14604, #17961, #21086, .T. ) ;
#9529=VECTOR ( 'NONE', #17762, 1000.000000000000114 ) ;
#9538=CARTESIAN_POINT ( 'NONE',  ( 1.342750202250000191, -63.28208324180000233, -144.5552959529999839 ) ) ;
#9540=CARTESIAN_POINT ( 'NONE',  ( -6.635402838469999232, -21.69968975860000171, -147.5552959529999839 ) ) ;
#9542=VECTOR ( 'NONE', #11585, 1000.000000000000000 ) ;
#9563=ORIENTED_EDGE ( 'NONE', *, *, #13997, .T. ) ;
#9565=LINE ( 'NONE', #13140, #3810 ) ;
#9571=ORIENTED_EDGE ( 'NONE', *, *, #1847, .F. ) ;
#9572=VECTOR ( 'NONE', #12341, 1000.000000000000114 ) ;
#9583=ORIENTED_EDGE ( 'NONE', *, *, #7340, .F. ) ;
#9593=VERTEX_POINT ( 'NONE', #3584 ) ;
#9600=ADVANCED_FACE ( 'NONE', ( #2048 ), #10812, .F. ) ;
#9603=ORIENTED_EDGE ( 'NONE', *, *, #497, .F. ) ;
#9606=CARTESIAN_POINT ( 'NONE',  ( 9.152949117179998595, -16.59780702190000312, -148.5552959529999839 ) ) ;
#9610=FACE_OUTER_BOUND ( 'NONE', #17472, .T. ) ;
#9612=ORIENTED_EDGE ( 'NONE', *, *, #8853, .T. ) ;
#9616=ORIENTED_EDGE ( 'NONE', *, *, #12301, .F. ) ;
#9618=LINE ( 'NONE', #6068, #14132 ) ;
#9620=ORIENTED_EDGE ( 'NONE', *, *, #18884, .T. ) ;
#9629=CARTESIAN_POINT ( 'NONE',  ( 23.19105773460000108, -15.44374190390000123, -145.5552959529999839 ) ) ;
#9631=DIRECTION ( 'NONE',  ( 0.000000000000000000, -1.000000000000000000, 8.159623473500000156E-13 ) ) ;
#9643=DIRECTION ( 'NONE',  ( -1.525446435830000185E-13, -8.171241461240000022E-13, -1.000000000000000000 ) ) ;
#9655=ADVANCED_FACE ( 'NONE', ( #14643 ), #11056, .F. ) ;
#9658=CARTESIAN_POINT ( 'NONE',  ( 24.89581725840000104, -26.85672394480000236, -143.5552959529999839 ) ) ;
#9669=ADVANCED_FACE ( 'NONE', ( #4049 ), #15344, .F. ) ;
#9676=ADVANCED_FACE ( 'NONE', ( #15104, #6290, #20816 ), #17125, .F. ) ;
#9682=CARTESIAN_POINT ( 'NONE',  ( 25.15155135439999867, -26.08415009650000016, -147.5552959529999839 ) ) ;
#9684=CARTESIAN_POINT ( 'NONE',  ( -6.635402838459999231, -21.69968975860000171, -146.5552959529999839 ) ) ;
#9685=ORIENTED_EDGE ( 'NONE', *, *, #11125, .T. ) ;
#9696=DIRECTION ( 'NONE',  ( 0.9988198443106121038, -0.04856869991388110958, -1.110673412899570175E-14 ) ) ;
#9698=DIRECTION ( 'NONE',  ( 0.2024296638729825848, 0.9792968044389154247, -3.587490878269691778E-13 ) ) ;
#9701=EDGE_CURVE ( 'NONE', #2580, #4564, #18443, .T. ) ;
#9712=ORIENTED_EDGE ( 'NONE', *, *, #23330, .T. ) ;
#9716=DIRECTION ( 'NONE',  ( -0.09606172499277226828, -0.9953753789357124848, 8.268372250837614805E-13 ) ) ;
#9719=DIRECTION ( 'NONE',  ( 1.526468026909999897E-13, 8.159623473500000156E-13, 1.000000000000000000 ) ) ;
#9725=DIRECTION ( 'NONE',  ( 2.842170943040000002E-14, 3.552713678800000097E-13, 1.000000000000000000 ) ) ;
#9729=CARTESIAN_POINT ( 'NONE',  ( 24.09267687515769296, -30.62512331353721251, -146.5552959530036503 ) ) ;
#9733=CARTESIAN_POINT ( 'NONE',  ( 15.97954986339999905, -26.72957102550000030, -143.5552959529999839 ) ) ;
#9736=VECTOR ( 'NONE', #3920, 999.9999999999998863 ) ;
#9741=CARTESIAN_POINT ( 'NONE',  ( -9.347107914279998653, -17.32706600430000066, -143.5552959529999839 ) ) ;
#9744=DIRECTION ( 'NONE',  ( 0.9991304227374304681, 0.04169410462551791791, -4.019436694231727866E-14 ) ) ;
#9753=DIRECTION ( 'NONE',  ( 0.9949850929136110356, -0.1000233216789610247, 7.446425804567098138E-15 ) ) ;
#9759=EDGE_CURVE ( 'NONE', #2337, #5226, #490, .T. ) ;
#9767=LINE ( 'NONE', #530, #2909 ) ;
#9772=DIRECTION ( 'NONE',  ( -0.09606172499277226828, -0.9953753789357124848, 8.268372250837614805E-13 ) ) ;
#9777=EDGE_CURVE ( 'NONE', #16462, #22505, #9377, .T. ) ;
#9778=ORIENTED_EDGE ( 'NONE', *, *, #14834, .F. ) ;
#9784=ORIENTED_EDGE ( 'NONE', *, *, #377, .T. ) ;
#9788=ORIENTED_EDGE ( 'NONE', *, *, #17660, .F. ) ;
#9801=ORIENTED_EDGE ( 'NONE', *, *, #9526, .F. ) ;
#9802=CARTESIAN_POINT ( 'NONE',  ( 15.87827223000000032, -26.60524292859999917, -144.0552959529999839 ) ) ;
#9822=AXIS2_PLACEMENT_3D ( 'NONE', #20546, #803, #22675 ) ;
#9826=AXIS2_PLACEMENT_3D ( 'NONE', #15209, #1049, #18885 ) ;
#9835=ORIENTED_EDGE ( 'NONE', *, *, #22549, .T. ) ;
#9847=ORIENTED_EDGE ( 'NONE', *, *, #4591, .T. ) ;
#9848=VECTOR ( 'NONE', #16237, 1000.000000000000000 ) ;
#9849=DIRECTION ( 'NONE',  ( 0.9915498581664488054, 0.1297261684090585954, -4.315191440381949291E-12 ) ) ;
#9858=ORIENTED_EDGE ( 'NONE', *, *, #21262, .T. ) ;
#9863=CIRCLE ( 'NONE', #3434, 6.000000000000001776 ) ;
#9865=DIRECTION ( 'NONE',  ( -0.1107105301439589573, -0.9938526945756315234, 8.278459860356925655E-13 ) ) ;
#9866=FACE_OUTER_BOUND ( 'NONE', #6060, .T. ) ;
#9870=CARTESIAN_POINT ( 'NONE',  ( 1.759100530420000030, -16.38142836440000139, -142.5552959529999839 ) ) ;
#9881=ORIENTED_EDGE ( 'NONE', *, *, #7210, .F. ) ;
#9887=DIRECTION ( 'NONE',  ( 1.526468026909999897E-13, 8.159623473500000156E-13, 1.000000000000000000 ) ) ;
#9892=CARTESIAN_POINT ( 'NONE',  ( 5.792747474889999637, -16.92794981449999980, -144.5552959529999839 ) ) ;
#9894=CIRCLE ( 'NONE', #3097, 8.176568160359998672 ) ;
#9897=EDGE_CURVE ( 'NONE', #20935, #1717, #15452, .T. ) ;
#9898=ORIENTED_EDGE ( 'NONE', *, *, #1065, .T. ) ;
#9906=DIRECTION ( 'NONE',  ( 8.955190032050000935E-12, -9.104778821549999739E-13, 1.000000000000000000 ) ) ;
#9911=AXIS2_PLACEMENT_3D ( 'NONE', #20056, #12314, #10754 ) ;
#9918=APPLICATION_CONTEXT ( 'automotive_design' ) ;
#9937=DIRECTION ( 'NONE',  ( 2.842170943040000002E-14, 3.552713678800000097E-13, 1.000000000000000000 ) ) ;
#9943=ORIENTED_EDGE ( 'NONE', *, *, #21704, .F. ) ;
#9952=EDGE_CURVE ( 'NONE', #22607, #760, #22840, .T. ) ;
#9959=DIRECTION ( 'NONE',  ( 0.9896415801065049367, -0.1435602414469282218, -8.993136838065500309E-12 ) ) ;
#9969=DIRECTION ( 'NONE',  ( -0.06206811009758109871, 0.9980719161006958995, -8.049146049297549005E-13 ) ) ;
#9971=CARTESIAN_POINT ( 'NONE',  ( -6.547730170579999509, -18.66441632429999942, -147.5552959529999839 ) ) ;
#9981=CARTESIAN_POINT ( 'NONE',  ( -8.916553640509999212, -11.88594259849999979, -143.5552959529999839 ) ) ;
#9983=ORIENTED_EDGE ( 'NONE', *, *, #5728, .F. ) ;
#9985=CARTESIAN_POINT ( 'NONE',  ( 7.228490359739999427, -13.33508289800000135, -145.5552959529999839 ) ) ;
#9988=LINE ( 'NONE', #19410, #7643 ) ;
#9989=CARTESIAN_POINT ( 'NONE',  ( -7.826190453620396781, -26.58762194555488989, -147.5552959530076009 ) ) ;
#9999=VECTOR ( 'NONE', #22079, 1000.000000000000000 ) ;
#10004=EDGE_CURVE ( 'NONE', #15489, #17671, #6757, .T. ) ;
#10007=ORIENTED_EDGE ( 'NONE', *, *, #3769, .F. ) ;
#10010=FACE_OUTER_BOUND ( 'NONE', #21382, .T. ) ;
#10013=CARTESIAN_POINT ( 'NONE',  ( 5.792747474879999636, -16.92794981449999980, -145.5552959529999839 ) ) ;
#10015=AXIS2_PLACEMENT_3D ( 'NONE', #12874, #18127, #1611 ) ;
#10016=ORIENTED_EDGE ( 'NONE', *, *, #14598, .T. ) ;
#10023=EDGE_LOOP ( 'NONE', ( #15549, #6024, #8591, #22429, #10260 ) ) ;
#10036=ORIENTED_EDGE ( 'NONE', *, *, #4924, .T. ) ;
#10038=EDGE_LOOP ( 'NONE', ( #18067, #20928, #19361, #11129, #12909, #17676, #7557 ) ) ;
#10040=ORIENTED_EDGE ( 'NONE', *, *, #4708, .F. ) ;
#10042=ORIENTED_EDGE ( 'NONE', *, *, #17578, .T. ) ;
#10045=ORIENTED_EDGE ( 'NONE', *, *, #4032, .T. ) ;
#10048=LINE ( 'NONE', #3065, #17074 ) ;
#10055=PLANE ( 'NONE',  #15528 ) ;
#10062=DIRECTION ( 'NONE',  ( -0.1000233216789610108, -0.9949850929136109245, 3.559993607998610461E-13 ) ) ;
#10067=ORIENTED_EDGE ( 'NONE', *, *, #3001, .F. ) ;
#10070=ORIENTED_EDGE ( 'NONE', *, *, #20012, .T. ) ;
#10073=VERTEX_POINT ( 'NONE', #16284 ) ;
#10080=PLANE ( 'NONE',  #1258 ) ;
#10081=ORIENTED_EDGE ( 'NONE', *, *, #21477, .F. ) ;
#10083=CARTESIAN_POINT ( 'NONE',  ( -6.165211177139999776, -15.11551140080000089, -143.0552959529999839 ) ) ;
#10084=EDGE_CURVE ( 'NONE', #2213, #6279, #3314, .T. ) ;
#10089=ORIENTED_EDGE ( 'NONE', *, *, #3052, .F. ) ;
#10098=ORIENTED_EDGE ( 'NONE', *, *, #17787, .F. ) ;
#10100=CIRCLE ( 'NONE', #11608, 14.99999999999999822 ) ;
#10104=LINE ( 'NONE', #19164, #14731 ) ;
#10107=ORIENTED_EDGE ( 'NONE', *, *, #6259, .T. ) ;
#10110=DIRECTION ( 'NONE',  ( 1.526468026909999897E-13, 8.159623473500000156E-13, 1.000000000000000000 ) ) ;
#10111=EDGE_CURVE ( 'NONE', #7689, #16462, #18416, .T. ) ;
#10116=ORIENTED_EDGE ( 'NONE', *, *, #12838, .T. ) ;
#10118=CARTESIAN_POINT ( 'NONE',  ( 19.86977406280000125, -31.59375768830000197, -147.5552959529999839 ) ) ;
#10123=PLANE ( 'NONE',  #7192 ) ;
#10128=LINE ( 'NONE', #19187, #20873 ) ;
#10134=VECTOR ( 'NONE', #5727, 1000.000000000000000 ) ;
#10135=( NAMED_UNIT ( * ) SI_UNIT ( $, .STERADIAN. ) SOLID_ANGLE_UNIT ( ) );
#10140=DIRECTION ( 'NONE',  ( 1.526468026909999897E-13, 8.159623473500000156E-13, 1.000000000000000000 ) ) ;
#10148=VECTOR ( 'NONE', #19012, 1000.000000000000000 ) ;
#10155=DIRECTION ( 'NONE',  ( 1.000000000000000000, 0.000000000000000000, -4.510774274160000731E-12 ) ) ;
#10162=VERTEX_POINT ( 'NONE', #20785 ) ;
#10169=PLANE ( 'NONE',  #17098 ) ;
#10180=PLANE ( 'NONE',  #13620 ) ;
#10183=VECTOR ( 'NONE', #21083, 1000.000000000000000 ) ;
#10186=DIRECTION ( 'NONE',  ( 0.9991304227374304681, 0.04169410462551791791, -4.421380363651902035E-14 ) ) ;
#10198=VERTEX_POINT ( 'NONE', #19354 ) ;
#10205=CARTESIAN_POINT ( 'NONE',  ( -8.594304764349999459, -10.75357442870000035, -145.0552959529999839 ) ) ;
#10213=CARTESIAN_POINT ( 'NONE',  ( 8.645354125658261779, -29.00058528980708417, -146.5552959529681232 ) ) ;
#10225=VECTOR ( 'NONE', #1640, 1000.000000000000114 ) ;
#10228=LINE ( 'NONE', #1221, #14129 ) ;
#10230=LINE ( 'NONE', #22734, #10183 ) ;
#10236=CARTESIAN_POINT ( 'NONE',  ( -4.521812268179999705, -27.38504028299999860, -148.0552959529999839 ) ) ;
#10238=ORIENTED_EDGE ( 'NONE', *, *, #15416, .F. ) ;
#10240=FACE_OUTER_BOUND ( 'NONE', #4934, .T. ) ;
#10241=ADVANCED_FACE ( 'NONE', ( #15423 ), #8399, .T. ) ;
#10243=EDGE_CURVE ( 'NONE', #19493, #1779, #8270, .T. ) ;
#10248=AXIS2_PLACEMENT_3D ( 'NONE', #16407, #1785, #21885 ) ;
#10250=VECTOR ( 'NONE', #21416, 1000.000000000000114 ) ;
#10253=EDGE_LOOP ( 'NONE', ( #8451, #10036, #9359, #11737, #21297, #10874 ) ) ;
#10256=DIRECTION ( 'NONE',  ( -0.9954742291034677226, 0.09503188512734457583, 4.503363594322118746E-12 ) ) ;
#10260=ORIENTED_EDGE ( 'NONE', *, *, #23166, .F. ) ;
#10268=MECHANICAL_DESIGN_GEOMETRIC_PRESENTATION_REPRESENTATION('',(#6857),#21305);
#10272=DIRECTION ( 'NONE',  ( 1.000000000000000000, 0.000000000000000000, -1.480297366166875808E-13 ) ) ;
#10283=EDGE_CURVE ( 'NONE', #20361, #10772, #10048, .T. ) ;
#10290=ORIENTED_EDGE ( 'NONE', *, *, #4133, .F. ) ;
#10291=ORIENTED_EDGE ( 'NONE', *, *, #177, .F. ) ;
#10294=ORIENTED_EDGE ( 'NONE', *, *, #12849, .T. ) ;
#10295=AXIS2_PLACEMENT_3D ( 'NONE', #10313, #22947, #6630 ) ;
#10298=DIRECTION ( 'NONE',  ( -0.07970438983373200059, -0.9968185442904001770, 8.268133652483321323E-13 ) ) ;
#10309=AXIS2_PLACEMENT_3D ( 'NONE', #13337, #9399, #11078 ) ;
#10313=CARTESIAN_POINT ( 'NONE',  ( -4.959431410700000598, -23.66636161550000139, -145.5552959529999839 ) ) ;
#10330=AXIS2_PLACEMENT_3D ( 'NONE', #5267, #12521, #23476 ) ;
#10335=EDGE_CURVE ( 'NONE', #8887, #15850, #5293, .T. ) ;
#10354=DIRECTION ( 'NONE',  ( -0.09606172499277226828, -0.9953753789357124848, 8.268372250837614805E-13 ) ) ;
#10359=EDGE_LOOP ( 'NONE', ( #10516, #22583, #3425, #16438 ) ) ;
#10362=PLANE ( 'NONE',  #19738 ) ;
#10367=LINE ( 'NONE', #6460, #10586 ) ;
#10368=ORIENTED_EDGE ( 'NONE', *, *, #6162, .T. ) ;
#10374=ORIENTED_EDGE ( 'NONE', *, *, #1847, .T. ) ;
#10380=EDGE_CURVE ( 'NONE', #4187, #11626, #5181, .T. ) ;
#10383=DIRECTION ( 'NONE',  ( 1.527666881879999979E-13, 8.153477892850000134E-13, 1.000000000000000000 ) ) ;
#10389=CYLINDRICAL_SURFACE ( 'NONE', #1524, 10.00000000000000178 ) ;
#10395=CARTESIAN_POINT ( 'NONE',  ( 8.212854026800000540, -28.22404483660000096, -144.5552959529999839 ) ) ;
#10404=DIRECTION ( 'NONE',  ( 1.526468026909999897E-13, 8.159623473500000156E-13, 1.000000000000000000 ) ) ;
#10405=ORIENTED_EDGE ( 'NONE', *, *, #4708, .T. ) ;
#10408=CIRCLE ( 'NONE', #8116, 9.999999999999998224 ) ;
#10416=CYLINDRICAL_SURFACE ( 'NONE', #13245, 5.000000000000000888 ) ;
#10436=DIRECTION ( 'NONE',  ( 8.955190032050000935E-12, -9.104778821549999739E-13, 1.000000000000000000 ) ) ;
#10439=CARTESIAN_POINT ( 'NONE',  ( 12.81474735470000148, -17.96536370379999781, -143.5552959529999839 ) ) ;
#10443=ORIENTED_EDGE ( 'NONE', *, *, #9433, .T. ) ;
#10451=PLANE ( 'NONE',  #18985 ) ;
#10452=CARTESIAN_POINT ( 'NONE',  ( 22.33963087269999903, -30.94765732060000119, -147.5552959529999839 ) ) ;
#10455=VECTOR ( 'NONE', #8721, 1000.000000000000000 ) ;
#10458=DIRECTION ( 'NONE',  ( -0.9896415801065049367, 0.1435602414469282218, 8.993136838065500309E-12 ) ) ;
#10463=EDGE_CURVE ( 'NONE', #16855, #8795, #16947, .T. ) ;
#10465=ORIENTED_EDGE ( 'NONE', *, *, #10111, .F. ) ;
#10466=FACE_OUTER_BOUND ( 'NONE', #20637, .T. ) ;
#10478=VERTEX_POINT ( 'NONE', #14695 ) ;
#10479=DIRECTION ( 'NONE',  ( -0.9753087663813413410, 0.2208456705930775810, 0.000000000000000000 ) ) ;
#10482=EDGE_CURVE ( 'NONE', #17961, #34, #1922, .T. ) ;
#10483=VERTEX_POINT ( 'NONE', #21964 ) ;
#10486=VECTOR ( 'NONE', #17423, 1000.000000000000114 ) ;
#10488=DIRECTION ( 'NONE',  ( -0.07970438983373200059, -0.9968185442904001770, 8.242295734823311485E-13 ) ) ;
#10495=CARTESIAN_POINT ( 'NONE',  ( -9.157754307290000284, -15.75963164970000108, -147.5552959529999839 ) ) ;
#10499=DIRECTION ( 'NONE',  ( 1.000000000000000000, 0.000000000000000000, -4.510774274160000731E-12 ) ) ;
#10503=DIRECTION ( 'NONE',  ( -0.9953753789357124848, 0.09606172499277215726, 7.216449660063520037E-14 ) ) ;
#10516=ORIENTED_EDGE ( 'NONE', *, *, #7770, .F. ) ;
#10524=ORIENTED_EDGE ( 'NONE', *, *, #23486, .F. ) ;
#10532=EDGE_CURVE ( 'NONE', #19961, #18313, #400, .T. ) ;
#10535=VECTOR ( 'NONE', #21428, 1000.000000000000000 ) ;
#10539=EDGE_CURVE ( 'NONE', #12475, #20935, #2214, .T. ) ;
#10541=CARTESIAN_POINT ( 'NONE',  ( -9.334216945200001447, -17.19633444960000190, -146.5552959529999839 ) ) ;
#10575=PLANE ( 'NONE',  #1563 ) ;
#10577=DIRECTION ( 'NONE',  ( 1.000000000000000000, 0.000000000000000000, -1.522591576628786004E-13 ) ) ;
#10579=CARTESIAN_POINT ( 'NONE',  ( -9.056357402059999728, -12.43025388040000045, -147.5552959529999839 ) ) ;
#10581=ORIENTED_EDGE ( 'NONE', *, *, #19294, .T. ) ;
#10586=VECTOR ( 'NONE', #21221, 1000.000000000000114 ) ;
#10588=ORIENTED_EDGE ( 'NONE', *, *, #14141, .F. ) ;
#10593=VECTOR ( 'NONE', #18533, 1000.000000000000114 ) ;
#10602=VERTEX_POINT ( 'NONE', #17300 ) ;
#10609=DIRECTION ( 'NONE',  ( -0.9874789572432817186, 0.1577507813030449846, 0.000000000000000000 ) ) ;
#10613=VECTOR ( 'NONE', #17976, 1000.000000000000000 ) ;
#10620=CARTESIAN_POINT ( 'NONE',  ( -9.394779979509999990, -17.86685386420000299, -143.5552959529999839 ) ) ;
#10626=EDGE_CURVE ( 'NONE', #15749, #22553, #12913, .T. ) ;
#10628=DIRECTION ( 'NONE',  ( -0.8020331419910812221, -0.5972795318340601289, 3.537910705138833522E-12 ) ) ;
#10629=AXIS2_PLACEMENT_3D ( 'NONE', #14091, #21714, #19804 ) ;
#10632=ORIENTED_EDGE ( 'NONE', *, *, #5745, .F. ) ;
#10645=AXIS2_PLACEMENT_3D ( 'NONE', #13925, #4884, #12131 ) ;
#10655=EDGE_CURVE ( 'NONE', #21497, #2284, #1548, .T. ) ;
#10656=EDGE_LOOP ( 'NONE', ( #1890, #121, #10443, #17154, #18123, #7713 ) ) ;
#10669=ORIENTED_EDGE ( 'NONE', *, *, #13273, .T. ) ;
#10677=EDGE_LOOP ( 'NONE', ( #4175, #10016, #9217, #14594 ) ) ;
#10682=EDGE_CURVE ( 'NONE', #3418, #2622, #2560, .T. ) ;
#10691=CARTESIAN_POINT ( 'NONE',  ( 8.633772787779999902, -29.00605602609999778, -147.0552959529999839 ) ) ;
#10693=DIRECTION ( 'NONE',  ( 4.518783361002970486E-12, 0.000000000000000000, 1.000000000000000000 ) ) ;
#10696=VECTOR ( 'NONE', #8879, 1000.000000000000227 ) ;
#10700=DIRECTION ( 'NONE',  ( 1.526468026909999897E-13, 8.159623473500000156E-13, 1.000000000000000000 ) ) ;
#10707=CARTESIAN_POINT ( 'NONE',  ( -9.434278515689999978, -18.41834002140000237, -147.5552959529999839 ) ) ;
#10708=EDGE_CURVE ( 'NONE', #3831, #5244, #22547, .T. ) ;
#10713=EDGE_LOOP ( 'NONE', ( #6845, #11178, #7217, #11466, #14958 ) ) ;
#10714=CIRCLE ( 'NONE', #97, 6.000000000000001776 ) ;
#10717=CARTESIAN_POINT ( 'NONE',  ( 22.27731556082403941, -15.33058227694559683, -144.5552959530006945 ) ) ;
#10725=CARTESIAN_POINT ( 'NONE',  ( 2.508811538190000245, -14.35090895149999923, -145.0552959529999839 ) ) ;
#10737=ORIENTED_EDGE ( 'NONE', *, *, #3717, .T. ) ;
#10742=CYLINDRICAL_SURFACE ( 'NONE', #3275, 3.000000000000000000 ) ;
#10747=CARTESIAN_POINT ( 'NONE',  ( 12.82492181439999968, -17.92284828160000032, -145.5552959529999839 ) ) ;
#10750=ORIENTED_EDGE ( 'NONE', *, *, #303, .F. ) ;
#10754=DIRECTION ( 'NONE',  ( 1.000000000000000000, 0.000000000000000000, -4.429789868254373788E-12 ) ) ;
#10762=DIRECTION ( 'NONE',  ( 4.123791986225375161E-10, 0.000000000000000000, -1.000000000000000000 ) ) ;
#10767=LINE ( 'NONE', #7097, #6032 ) ;
#10772=VERTEX_POINT ( 'NONE', #12177 ) ;
#10785=LINE ( 'NONE', #3202, #9572 ) ;
#10804=DIRECTION ( 'NONE',  ( 1.000000000000000000, 0.000000000000000000, -1.498801083243961330E-13 ) ) ;
#10807=DIRECTION ( 'NONE',  ( 2.839308199620000013E-14, 3.568879590630000244E-13, 1.000000000000000000 ) ) ;
#10812=PLANE ( 'NONE',  #1884 ) ;
#10813=ADVANCED_FACE ( 'NONE', ( #23251 ), #14319, .T. ) ;
#10816=CARTESIAN_POINT ( 'NONE',  ( 1.829659965300000080, -16.02499107890000118, -144.0552959529999839 ) ) ;
#10821=EDGE_CURVE ( 'NONE', #1892, #22553, #3497, .T. ) ;
#10823=ORIENTED_EDGE ( 'NONE', *, *, #17238, .T. ) ;
#10824=EDGE_CURVE ( 'NONE', #2894, #14227, #22813, .T. ) ;
#10830=ORIENTED_EDGE ( 'NONE', *, *, #3769, .T. ) ;
#10842=ORIENTED_EDGE ( 'NONE', *, *, #15785, .T. ) ;
#10850=CIRCLE ( 'NONE', #13909, 35.00000000000000000 ) ;
#10851=VERTEX_POINT ( 'NONE', #17275 ) ;
#10852=LINE ( 'NONE', #19679, #1175 ) ;
#10858=CARTESIAN_POINT ( 'NONE',  ( -9.282104535849999394, -16.71402168319999859, -144.5552959529999839 ) ) ;
#10866=EDGE_CURVE ( 'NONE', #10483, #2706, #4781, .T. ) ;
#10871=VERTEX_POINT ( 'NONE', #22631 ) ;
#10874=ORIENTED_EDGE ( 'NONE', *, *, #7065, .F. ) ;
#10876=ORIENTED_EDGE ( 'NONE', *, *, #7117, .F. ) ;
#10884=DIRECTION ( 'NONE',  ( -0.1435602414469281940, -0.9896415801065048257, 3.836930773098079160E-13 ) ) ;
#10887=CARTESIAN_POINT ( 'NONE',  ( 16.25412235410000150, -22.59491385829999999, -146.5552959529999839 ) ) ;
#10888=ORIENTED_EDGE ( 'NONE', *, *, #21483, .T. ) ;
#10890=ADVANCED_FACE ( 'NONE', ( #22988 ), #3914, .F. ) ;
#10892=ORIENTED_EDGE ( 'NONE', *, *, #18244, .F. ) ;
#10893=ADVANCED_FACE ( 'NONE', ( #13936 ), #21533, .T. ) ;
#10895=AXIS2_PLACEMENT_3D ( 'NONE', #17908, #6714, #13976 ) ;
#10898=ORIENTED_EDGE ( 'NONE', *, *, #21483, .F. ) ;
#10913=PLANE ( 'NONE',  #9065 ) ;
#10917=EDGE_CURVE ( 'NONE', #14032, #4852, #14065, .T. ) ;
#10923=CARTESIAN_POINT ( 'NONE',  ( 16.64676602990000021, -18.64223989710000140, -143.5552959529999839 ) ) ;
#10924=PLANE ( 'NONE',  #14476 ) ;
#10929=DIRECTION ( 'NONE',  ( 1.000000000000000000, 0.000000000000000000, -1.527536832333223921E-13 ) ) ;
#10934=EDGE_CURVE ( 'NONE', #1717, #4754, #16345, .T. ) ;
#10939=CARTESIAN_POINT ( 'NONE',  ( 16.25412235410000150, -22.59491385829999999, -145.5552959529999839 ) ) ;
#10944=ORIENTED_EDGE ( 'NONE', *, *, #20315, .F. ) ;
#10950=DIRECTION ( 'NONE',  ( 9.087266560786239640E-12, 0.000000000000000000, 1.000000000000000000 ) ) ;
#10956=DIRECTION ( 'NONE',  ( -0.9694775522152123681, 0.2451800884060535979, 8.905086759541945709E-12 ) ) ;
#10958=AXIS2_PLACEMENT_3D ( 'NONE', #7123, #9129, #1672 ) ;
#10962=EDGE_CURVE ( 'NONE', #19736, #1038, #3675, .T. ) ;
#10967=ORIENTED_EDGE ( 'NONE', *, *, #22277, .F. ) ;
#10972=VECTOR ( 'NONE', #4893, 1000.000000000000114 ) ;
#10974=VECTOR ( 'NONE', #3800, 1000.000000000000000 ) ;
#10984=CARTESIAN_POINT ( 'NONE',  ( 22.11021350718841560, -15.30096212033725322, -145.5552959529996997 ) ) ;
#10990=VECTOR ( 'NONE', #9937, 1000.000000000000000 ) ;
#10992=ORIENTED_EDGE ( 'NONE', *, *, #10708, .T. ) ;
#10998=ORIENTED_EDGE ( 'NONE', *, *, #14269, .F. ) ;
#11003=FACE_OUTER_BOUND ( 'NONE', #20818, .T. ) ;
#11025=VERTEX_POINT ( 'NONE', #20330 ) ;
#11029=ORIENTED_EDGE ( 'NONE', *, *, #10934, .T. ) ;
#11031=LINE ( 'NONE', #6790, #2006 ) ;
#11041=AXIS2_PLACEMENT_3D ( 'NONE', #10725, #23473, #3490 ) ;
#11042=CARTESIAN_POINT ( 'NONE',  ( -8.734077015120000453, -11.22642389220000148, -146.0552959529999839 ) ) ;
#11056=CYLINDRICAL_SURFACE ( 'NONE', #17836, 35.00000000000000000 ) ;
#11058=DIRECTION ( 'NONE',  ( 2.839308199620000013E-14, 3.568879590630000244E-13, 1.000000000000000000 ) ) ;
#11071=DIRECTION ( 'NONE',  ( 0.4108698089121693986, -0.9116940276893763517, 3.145631903104610871E-13 ) ) ;
#11072=ORIENTED_EDGE ( 'NONE', *, *, #22608, .F. ) ;
#11078=DIRECTION ( 'NONE',  ( 0.000000000000000000, -1.000000000000000000, 8.159623473500000156E-13 ) ) ;
#11083=PLANE ( 'NONE',  #12216 ) ;
#11084=DIRECTION ( 'NONE',  ( 1.526468026909999897E-13, 8.159623473500000156E-13, 1.000000000000000000 ) ) ;
#11087=VECTOR ( 'NONE', #16040, 1000.000000000000227 ) ;
#11088=AXIS2_PLACEMENT_3D ( 'NONE', #23220, #1338, #14290 ) ;
#11099=DIRECTION ( 'NONE',  ( -0.1297261684090585954, 0.9915498581664488054, 1.179599313710532933E-12 ) ) ;
#11119=EDGE_LOOP ( 'NONE', ( #3195, #17715, #16625, #11398, #3687 ) ) ;
#11125=EDGE_CURVE ( 'NONE', #18387, #5495, #2822, .T. ) ;
#11127=ORIENTED_EDGE ( 'NONE', *, *, #3740, .T. ) ;
#11129=ORIENTED_EDGE ( 'NONE', *, *, #7770, .T. ) ;
#11131=EDGE_CURVE ( 'NONE', #15988, #18172, #1045, .T. ) ;
#11132=ORIENTED_EDGE ( 'NONE', *, *, #14085, .F. ) ;
#11136=FACE_OUTER_BOUND ( 'NONE', #13606, .T. ) ;
#11162=DIRECTION ( 'NONE',  ( 4.510774274160000731E-12, -1.321907670990000086E-13, 1.000000000000000000 ) ) ;
#11165=CARTESIAN_POINT ( 'NONE',  ( -6.334350183781824128, -17.33929910105837990, -144.5552959530011208 ) ) ;
#11172=CARTESIAN_POINT ( 'NONE',  ( 22.33963087269999903, -30.94765732060000119, -147.5552959529999839 ) ) ;
#11175=VECTOR ( 'NONE', #11905, 999.9999999999998863 ) ;
#11178=ORIENTED_EDGE ( 'NONE', *, *, #2562, .T. ) ;
#11179=ORIENTED_EDGE ( 'NONE', *, *, #10824, .T. ) ;
#11180=CARTESIAN_POINT ( 'NONE',  ( -9.434278515689999978, -18.41834002140000237, -147.5552959529999839 ) ) ;
#11182=CARTESIAN_POINT ( 'NONE',  ( 25.15155135439999867, -26.08415009650000016, -146.5552959529999839 ) ) ;
#11192=EDGE_CURVE ( 'NONE', #15113, #5364, #12792, .T. ) ;
#11199=ORIENTED_EDGE ( 'NONE', *, *, #4351, .T. ) ;
#11200=FILL_AREA_STYLE ('',( #21944 ) ) ;
#11215=ORIENTED_EDGE ( 'NONE', *, *, #2645, .F. ) ;
#11237=EDGE_CURVE ( 'NONE', #2622, #17961, #5351, .T. ) ;
#11246=VERTEX_POINT ( 'NONE', #21505 ) ;
#11251=CARTESIAN_POINT ( 'NONE',  ( -4.888913597060000171, -24.24628707910000003, -143.5552959529999839 ) ) ;
#11252=DIRECTION ( 'NONE',  ( -0.1435602414469281940, -0.9896415801065048257, 3.849849731938073961E-13 ) ) ;
#11253=ADVANCED_FACE ( 'NONE', ( #8867 ), #23399, .T. ) ;
#11258=EDGE_CURVE ( 'NONE', #22422, #7225, #7331, .T. ) ;
#11263=EDGE_CURVE ( 'NONE', #10478, #6817, #13257, .T. ) ;
#11269=VECTOR ( 'NONE', #18605, 1000.000000000000227 ) ;
#11270=ORIENTED_EDGE ( 'NONE', *, *, #13746, .F. ) ;
#11282=CARTESIAN_POINT ( 'NONE',  ( -9.347107914279998653, -17.32706600430000066, -143.5552959529999839 ) ) ;
#11283=PLANE ( 'NONE',  #7305 ) ;
#11289=LINE ( 'NONE', #15353, #13605 ) ;
#11290=ORIENTED_EDGE ( 'NONE', *, *, #5613, .F. ) ;
#11292=ORIENTED_EDGE ( 'NONE', *, *, #7650, .F. ) ;
#11299=FACE_OUTER_BOUND ( 'NONE', #7227, .T. ) ;
#11319=DIRECTION ( 'NONE',  ( -1.526468026909999897E-13, -8.159623473500000156E-13, -1.000000000000000000 ) ) ;
#11325=CARTESIAN_POINT ( 'NONE',  ( 24.59017985859999911, -26.91621017459999976, -148.5552959529999839 ) ) ;
#11326=DIRECTION ( 'NONE',  ( 4.511946372079999833E-12, -1.278976924369999890E-13, 1.000000000000000000 ) ) ;
#11334=DIRECTION ( 'NONE',  ( 0.000000000000000000, -1.000000000000000000, 8.159623473500000156E-13 ) ) ;
#11338=VECTOR ( 'NONE', #14648, 1000.000000000000227 ) ;
#11341=ORIENTED_EDGE ( 'NONE', *, *, #2533, .F. ) ;
#11347=CARTESIAN_POINT ( 'NONE',  ( -5.758148842630000708, -13.22138763369999914, -148.0552959529999839 ) ) ;
#11351=AXIS2_PLACEMENT_3D ( 'NONE', #4128, #13400, #811 ) ;
#11352=VECTOR ( 'NONE', #16404, 1000.000000000000114 ) ;
#11353=AXIS2_PLACEMENT_3D ( 'NONE', #19979, #16630, #5467 ) ;
#11365=AXIS2_PLACEMENT_3D ( 'NONE', #6862, #7337, #16149 ) ;
#11369=CARTESIAN_POINT ( 'NONE',  ( 6.841811532410000396, -13.03968765259999962, -145.5552959529999839 ) ) ;
#11375=VECTOR ( 'NONE', #18436, 1000.000000000000227 ) ;
#11380=CARTESIAN_POINT ( 'NONE',  ( 8.212854026790001427, -28.22404483660000096, -145.0552959529999839 ) ) ;
#11398=ORIENTED_EDGE ( 'NONE', *, *, #18752, .T. ) ;
#11404=EDGE_CURVE ( 'NONE', #1427, #13434, #17305, .T. ) ;
#11405=DIRECTION ( 'NONE',  ( -0.9954742291034677226, 0.09503188512734457583, 4.503363594322118746E-12 ) ) ;
#11410=ADVANCED_FACE ( 'NONE', ( #1492 ), #9189, .F. ) ;
#11412=EDGE_LOOP ( 'NONE', ( #19885, #370, #7755 ) ) ;
#11419=FACE_OUTER_BOUND ( 'NONE', #20179, .T. ) ;
#11439=VERTEX_POINT ( 'NONE', #21832 ) ;
#11443=DIRECTION ( 'NONE',  ( 1.000000000000000000, 0.000000000000000000, -4.430318231639999944E-12 ) ) ;
#11448=CARTESIAN_POINT ( 'NONE',  ( 8.212854026790001427, -28.22404483660000096, -145.5552959529999839 ) ) ;
#11453=VERTEX_POINT ( 'NONE', #12765 ) ;
#11455=ADVANCED_FACE ( 'NONE', ( #5516 ), #12651, .T. ) ;
#11458=FACE_OUTER_BOUND ( 'NONE', #5609, .T. ) ;
#11459=CIRCLE ( 'NONE', #22115, 35.00000000000000000 ) ;
#11460=AXIS2_PLACEMENT_3D ( 'NONE', #23248, #3369, #17892 ) ;
#11462=AXIS2_PLACEMENT_3D ( 'NONE', #8454, #1101, #19291 ) ;
#11466=ORIENTED_EDGE ( 'NONE', *, *, #5149, .T. ) ;
#11475=DIRECTION ( 'NONE',  ( 4.430318231639999944E-12, -6.100259101500000139E-13, 1.000000000000000000 ) ) ;
#11477=DIRECTION ( 'NONE',  ( 1.527666881879999979E-13, 8.171241461240000022E-13, 1.000000000000000000 ) ) ;
#11479=ORIENTED_EDGE ( 'NONE', *, *, #21188, .F. ) ;
#11482=EDGE_LOOP ( 'NONE', ( #2365, #9858, #2810 ) ) ;
#11485=VERTEX_POINT ( 'NONE', #14094 ) ;
#11486=EDGE_LOOP ( 'NONE', ( #14845, #21473, #4996, #20200 ) ) ;
#11501=EDGE_LOOP ( 'NONE', ( #13929, #15360, #5053, #518, #10290, #9801 ) ) ;
#11506=CYLINDRICAL_SURFACE ( 'NONE', #7581, 8.176568160360002224 ) ;
#11508=ORIENTED_EDGE ( 'NONE', *, *, #8137, .T. ) ;
#11516=VERTEX_POINT ( 'NONE', #12404 ) ;
#11519=CARTESIAN_POINT ( 'NONE',  ( 1.172620240290000115, -63.19354141059999108, -146.5552959529999839 ) ) ;
#11522=EDGE_CURVE ( 'NONE', #22098, #2580, #10852, .T. ) ;
#11529=PLANE ( 'NONE',  #23468 ) ;
#11536=PLANE ( 'NONE',  #12593 ) ;
#11538=MANIFOLD_SOLID_BREP ( 'lock_assembly.1\\Part8.1.2\\PartBody', #16777 ) ;
#11544=DIRECTION ( 'NONE',  ( 0.9949850929136110356, -0.1000233216789610247, 7.446425804567098138E-15 ) ) ;
#11545=VERTEX_POINT ( 'NONE', #9411 ) ;
#11585=DIRECTION ( 'NONE',  ( -0.1435602414469281940, -0.9896415801065048257, 3.836930773098079160E-13 ) ) ;
#11588=DIRECTION ( 'NONE',  ( -0.1577507813030449846, -0.9874789572432817186, 8.298258002992369366E-13 ) ) ;
#11589=VECTOR ( 'NONE', #13975, 1000.000000000000000 ) ;
#11590=VERTEX_POINT ( 'NONE', #14795 ) ;
#11600=CARTESIAN_POINT ( 'NONE',  ( 16.65835875212643913, -18.90326720743800593, -147.5552959530498640 ) ) ;
#11602=CARTESIAN_POINT ( 'NONE',  ( -6.370493725020000220, -17.65251768590000125, -145.5552959529999839 ) ) ;
#11608=AXIS2_PLACEMENT_3D ( 'NONE', #21219, #12273, #4793 ) ;
#11615=CARTESIAN_POINT ( 'NONE',  ( 15.87827223000000032, -26.60524292859999917, -144.5552959529999839 ) ) ;
#11618=DIRECTION ( 'NONE',  ( 0.000000000000000000, -1.000000000000000000, 8.159623473500000156E-13 ) ) ;
#11623=ORIENTED_EDGE ( 'NONE', *, *, #22849, .T. ) ;
#11626=VERTEX_POINT ( 'NONE', #9540 ) ;
#11636=DIRECTION ( 'NONE',  ( -0.1000233216789610108, -0.9949850929136109245, 3.559993607998610461E-13 ) ) ;
#11639=ADVANCED_FACE ( 'NONE', ( #2188 ), #405, .T. ) ;
#11649=FACE_OUTER_BOUND ( 'NONE', #11486, .T. ) ;
#11663=LINE ( 'NONE', #4203, #2776 ) ;
#11664=CARTESIAN_POINT ( 'NONE',  ( 22.42370904790000097, -21.41421288319999761, -143.0552959529999839 ) ) ;
#11669=CARTESIAN_POINT ( 'NONE',  ( -8.734077015120000453, -11.22642389220000148, -145.5552959529999839 ) ) ;
#11675=CARTESIAN_POINT ( 'NONE',  ( 2.170391987449999505, -12.72823260819999902, -146.0552959529999839 ) ) ;
#11685=DIRECTION ( 'NONE',  ( -0.9980143568310856361, 0.06298685227120542907, 4.509810669690391193E-12 ) ) ;
#11704=VECTOR ( 'NONE', #12254, 1000.000000000000000 ) ;
#11737=ORIENTED_EDGE ( 'NONE', *, *, #2419, .T. ) ;
#11739=DIRECTION ( 'NONE',  ( -1.527666881879999979E-13, -8.171241461240000022E-13, -1.000000000000000000 ) ) ;
#11753=LINE ( 'NONE', #9971, #16349 ) ;
#11754=EDGE_LOOP ( 'NONE', ( #5343, #14948, #4433, #3261 ) ) ;
#11769=CARTESIAN_POINT ( 'NONE',  ( 1.847645635000000119, -15.93876195360000025, -146.0552959529999839 ) ) ;
#11772=FACE_OUTER_BOUND ( 'NONE', #1526, .T. ) ;
#11780=DIRECTION ( 'NONE',  ( 1.000000000000000000, 0.000000000000000000, -1.480297366166875808E-13 ) ) ;
#11781=EDGE_CURVE ( 'NONE', #3115, #10871, #23123, .T. ) ;
#11786=DIRECTION ( 'NONE',  ( 1.527666881879999979E-13, 8.153477892850000134E-13, 1.000000000000000000 ) ) ;
#11793=ORIENTED_EDGE ( 'NONE', *, *, #12838, .F. ) ;
#11801=LINE ( 'NONE', #7766, #16924 ) ;
#11812=ORIENTED_EDGE ( 'NONE', *, *, #2645, .T. ) ;
#11816=AXIS2_PLACEMENT_3D ( 'NONE', #18863, #8697, #7047 ) ;
#11825=CYLINDRICAL_SURFACE ( 'NONE', #2181, 4.999999999999998224 ) ;
#11826=ADVANCED_FACE ( 'NONE', ( #23361 ), #5392, .T. ) ;
#11842=DIRECTION ( 'NONE',  ( 0.000000000000000000, -1.000000000000000000, 8.159623473500000156E-13 ) ) ;
#11850=CARTESIAN_POINT ( 'NONE',  ( -9.434278515689999978, -18.41834002140000237, -146.5552959529999839 ) ) ;
#11852=EDGE_CURVE ( 'NONE', #9023, #473, #1956, .T. ) ;
#11861=DIRECTION ( 'NONE',  ( 4.430318231639999944E-12, -6.100259101500000139E-13, 1.000000000000000000 ) ) ;
#11877=DIRECTION ( 'NONE',  ( 0.4860683305472111027, 0.8739208076473790054, -3.557471777477465713E-12 ) ) ;
#11879=PLANE ( 'NONE',  #5319 ) ;
#11893=CARTESIAN_POINT ( 'NONE',  ( -9.434278515689999978, -18.41834002140000237, -146.5552959529999839 ) ) ;
#11902=LINE ( 'NONE', #21087, #5013 ) ;
#11905=DIRECTION ( 'NONE',  ( -0.9954742291034677226, 0.09503188512734457583, 4.503697062742119365E-12 ) ) ;
#11908=DIRECTION ( 'NONE',  ( 0.9968185442904002880, -0.07970438983373201447, -8.712538262633510059E-14 ) ) ;
#11911=EDGE_LOOP ( 'NONE', ( #3761, #19564, #21427, #16500, #15068 ) ) ;
#11927=VERTEX_POINT ( 'NONE', #16562 ) ;
#11934=CARTESIAN_POINT ( 'NONE',  ( 22.42370904790000097, -21.41421288319999761, -143.5552959529999839 ) ) ;
#11969=CARTESIAN_POINT ( 'NONE',  ( -9.157754307290000284, -15.75963164970000108, -147.5552959529999839 ) ) ;
#11982=CARTESIAN_POINT ( 'NONE',  ( 2.068499633510000102, -14.99362786250000035, -147.5552959529999839 ) ) ;
#11995=VERTEX_POINT ( 'NONE', #8209 ) ;
#11996=VECTOR ( 'NONE', #10256, 999.9999999999998863 ) ;
#11997=FACE_OUTER_BOUND ( 'NONE', #14247, .T. ) ;
#12000=DIRECTION ( 'NONE',  ( -0.9847555042252370550, 0.1739442350240419932, 1.095575354920264064E-14 ) ) ;
#12003=ORIENTED_EDGE ( 'NONE', *, *, #10539, .F. ) ;
#12006=VERTEX_POINT ( 'NONE', #2876 ) ;
#12010=PLANE ( 'NONE',  #14037 ) ;
#12011=VECTOR ( 'NONE', #4875, 1000.000000000000000 ) ;
#12015=CARTESIAN_POINT ( 'NONE',  ( 5.792747474879999636, -16.92794981449999980, -145.5552959529999839 ) ) ;
#12022=DIRECTION ( 'NONE',  ( 1.526468026909999897E-13, 8.159623473500000156E-13, 1.000000000000000000 ) ) ;
#12034=ORIENTED_EDGE ( 'NONE', *, *, #14217, .F. ) ;
#12041=LINE ( 'NONE', #17884, #2506 ) ;
#12062=FACE_OUTER_BOUND ( 'NONE', #7841, .T. ) ;
#12067=ORIENTED_EDGE ( 'NONE', *, *, #16098, .T. ) ;
#12072=ORIENTED_EDGE ( 'NONE', *, *, #13409, .F. ) ;
#12079=EDGE_CURVE ( 'NONE', #20700, #22206, #21738, .T. ) ;
#12089=VECTOR ( 'NONE', #29, 1000.000000000000000 ) ;
#12092=DIRECTION ( 'NONE',  ( -0.1000233216789610108, -0.9949850929136109245, 3.591470555298595137E-13 ) ) ;
#12094=CIRCLE ( 'NONE', #17438, 35.00000000000000000 ) ;
#12095=DIRECTION ( 'NONE',  ( -0.9753087663813413410, 0.2208456705930775810, 8.935806277123132252E-12 ) ) ;
#12099=EDGE_CURVE ( 'NONE', #23414, #4587, #17980, .T. ) ;
#12106=ORIENTED_EDGE ( 'NONE', *, *, #16732, .F. ) ;
#12114=CARTESIAN_POINT ( 'NONE',  ( 24.11847952820000174, -31.58456057200000089, -143.5552959529999839 ) ) ;
#12127=PLANE ( 'NONE',  #9009 ) ;
#12131=DIRECTION ( 'NONE',  ( 0.000000000000000000, -1.000000000000000000, 3.568879590630000244E-13 ) ) ;
#12146=FACE_OUTER_BOUND ( 'NONE', #12591, .T. ) ;
#12155=VERTEX_POINT ( 'NONE', #9024 ) ;
#12159=CARTESIAN_POINT ( 'NONE',  ( 22.32684911886484613, -15.33692515329977546, -144.5552959530006945 ) ) ;
#12163=FACE_OUTER_BOUND ( 'NONE', #674, .T. ) ;
#12167=ORIENTED_EDGE ( 'NONE', *, *, #5142, .T. ) ;
#12170=AXIS2_PLACEMENT_3D ( 'NONE', #5276, #19921, #1730 ) ;
#12175=CARTESIAN_POINT ( 'NONE',  ( -4.521812268189999706, -27.38504028299999860, -148.5552959529999839 ) ) ;
#12176=ORIENTED_EDGE ( 'NONE', *, *, #17107, .T. ) ;
#12177=CARTESIAN_POINT ( 'NONE',  ( -7.002253344594251416, -25.58393298470214816, -143.5552959529972554 ) ) ;
#12184=DIRECTION ( 'NONE',  ( 0.000000000000000000, -1.000000000000000000, 8.159623473500000156E-13 ) ) ;
#12191=ORIENTED_EDGE ( 'NONE', *, *, #10532, .T. ) ;
#12207=FACE_OUTER_BOUND ( 'NONE', #22500, .T. ) ;
#12216=AXIS2_PLACEMENT_3D ( 'NONE', #18362, #22276, #20379 ) ;
#12217=AXIS2_PLACEMENT_3D ( 'NONE', #16252, #14690, #1986 ) ;
#12220=EDGE_LOOP ( 'NONE', ( #22031, #19699, #9489, #15160, #8819, #2288, #922 ) ) ;
#12228=DIRECTION ( 'NONE',  ( 1.527666881879999979E-13, 8.171241461240000022E-13, 1.000000000000000000 ) ) ;
#12229=ORIENTED_EDGE ( 'NONE', *, *, #3157, .T. ) ;
#12231=DIRECTION ( 'NONE',  ( -0.07970438983373200059, -0.9968185442904001770, 8.242295734823311485E-13 ) ) ;
#12239=CARTESIAN_POINT ( 'NONE',  ( -8.770737564319999180, -11.35481373070000011, -144.5552959529999839 ) ) ;
#12242=CARTESIAN_POINT ( 'NONE',  ( 15.85402906740000084, -26.57485422999999969, -145.5552959529999839 ) ) ;
#12252=CARTESIAN_POINT ( 'NONE',  ( 17.45728951470000112, -20.98759093920000041, -146.5552959529999839 ) ) ;
#12254=DIRECTION ( 'NONE',  ( 1.527666881879999979E-13, 8.171241461240000022E-13, 1.000000000000000000 ) ) ;
#12262=LINE ( 'NONE', #15960, #16121 ) ;
#12266=ORIENTED_EDGE ( 'NONE', *, *, #109, .T. ) ;
#12267=EDGE_CURVE ( 'NONE', #10772, #13630, #1389, .T. ) ;
#12271=LINE ( 'NONE', #15971, #18592 ) ;
#12273=DIRECTION ( 'NONE',  ( 4.510774274160000731E-12, -1.321907670990000086E-13, 1.000000000000000000 ) ) ;
#12274=CARTESIAN_POINT ( 'NONE',  ( 17.66940543669999997, -18.68690163239999791, -145.5552959529999839 ) ) ;
#12282=CARTESIAN_POINT ( 'NONE',  ( -6.477935707790000386, -19.20465386649999928, -147.5552959529999839 ) ) ;
#12285=EDGE_CURVE ( 'NONE', #14669, #1892, #19478, .T. ) ;
#12291=VERTEX_POINT ( 'NONE', #15889 ) ;
#12297=CARTESIAN_POINT ( 'NONE',  ( 2.139623390130000136, -12.81320239329999922, -143.5552959529999839 ) ) ;
#12301=EDGE_CURVE ( 'NONE', #16939, #5364, #4231, .T. ) ;
#12314=DIRECTION ( 'NONE',  ( 4.430318231639999944E-12, -6.100259101500000139E-13, 1.000000000000000000 ) ) ;
#12322=EDGE_LOOP ( 'NONE', ( #14427, #18470, #19232, #3323, #19725 ) ) ;
#12330=PLANE ( 'NONE',  #23114 ) ;
#12338=EDGE_LOOP ( 'NONE', ( #16292, #667, #12034 ) ) ;
#12341=DIRECTION ( 'NONE',  ( -0.06298685227120542907, -0.9980143568310855251, 1.515824502950130739E-13 ) ) ;
#12342=ORIENTED_EDGE ( 'NONE', *, *, #5613, .T. ) ;
#12345=CARTESIAN_POINT ( 'NONE',  ( 12.94820732169999999, -17.45719265660000019, -147.5552959529999839 ) ) ;
#12348=VECTOR ( 'NONE', #619, 1000.000000000000000 ) ;
#12350=ORIENTED_EDGE ( 'NONE', *, *, #8881, .F. ) ;
#12352=DIRECTION ( 'NONE',  ( -0.9913873220698726785, 0.1309625047069831461, -1.853446743629759619E-14 ) ) ;
#12355=CARTESIAN_POINT ( 'NONE',  ( 6.477506801250000557, -13.91317765220000169, -146.5552959529999839 ) ) ;
#12374=CARTESIAN_POINT ( 'NONE',  ( -9.334216945200001447, -17.19633444960000190, -145.5552959529999839 ) ) ;
#12385=CARTESIAN_POINT ( 'NONE',  ( 23.41308733940000053, -15.43505800149999985, -147.5552959529999839 ) ) ;
#12396=CARTESIAN_POINT ( 'NONE',  ( -6.599319970649999867, -19.98386714700000155, -146.5552959529999839 ) ) ;
#12401=DIRECTION ( 'NONE',  ( 0.9988198443106121038, -0.04856869991388110958, -1.110673412899570175E-14 ) ) ;
#12404=CARTESIAN_POINT ( 'NONE',  ( 8.982728679470000088, -17.28848751049999777, -143.5552959529999839 ) ) ;
#12408=VECTOR ( 'NONE', #8928, 1000.000000000000000 ) ;
#12410=ADVANCED_FACE ( 'NONE', ( #7428 ), #7086, .T. ) ;
#12415=LINE ( 'NONE', #9075, #20799 ) ;
#12417=ORIENTED_EDGE ( 'NONE', *, *, #21475, .F. ) ;
#12422=ORIENTED_EDGE ( 'NONE', *, *, #5333, .F. ) ;
#12444=DIRECTION ( 'NONE',  ( 2.839308199620000013E-14, 3.568879590630000244E-13, 1.000000000000000000 ) ) ;
#12448=DIRECTION ( 'NONE',  ( 4.430233957459999899E-12, -6.110667527539999876E-13, 1.000000000000000000 ) ) ;
#12451=ORIENTED_EDGE ( 'NONE', *, *, #21006, .T. ) ;
#12459=ORIENTED_EDGE ( 'NONE', *, *, #18941, .T. ) ;
#12462=ORIENTED_EDGE ( 'NONE', *, *, #10380, .F. ) ;
#12463=DIRECTION ( 'NONE',  ( -0.9954742291034677226, 0.09503188512734457583, 4.503697062742119365E-12 ) ) ;
#12464=DIRECTION ( 'NONE',  ( 1.000000000000000000, 0.000000000000000000, -2.854859206178974232E-14 ) ) ;
#12475=VERTEX_POINT ( 'NONE', #12872 ) ;
#12479=LINE ( 'NONE', #14744, #19796 ) ;
#12482=ADVANCED_FACE ( 'NONE', ( #14561 ), #12756, .F. ) ;
#12483=CARTESIAN_POINT ( 'NONE',  ( -9.334216945200001447, -17.19633444960000190, -145.5552959529999839 ) ) ;
#12495=CARTESIAN_POINT ( 'NONE',  ( 16.25412235410000150, -22.59491385829999999, -146.5552959529999839 ) ) ;
#12498=VECTOR ( 'NONE', #4266, 999.9999999999998863 ) ;
#12506=LINE ( 'NONE', #1708, #12408 ) ;
#12513=EDGE_CURVE ( 'NONE', #9187, #4619, #3493, .T. ) ;
#12517=CIRCLE ( 'NONE', #11365, 35.00000000000000000 ) ;
#12518=AXIS2_PLACEMENT_3D ( 'NONE', #5608, #13332, #11071 ) ;
#12520=CARTESIAN_POINT ( 'NONE',  ( -9.334216945200001447, -17.19633444960000190, -146.5552959529999839 ) ) ;
#12521=DIRECTION ( 'NONE',  ( 4.430318231639999944E-12, -6.100259101500000139E-13, 1.000000000000000000 ) ) ;
#12526=DIRECTION ( 'NONE',  ( 0.1146332952500066227, 0.9934078757590583120, 9.947598300640582187E-14 ) ) ;
#12527=ORIENTED_EDGE ( 'NONE', *, *, #19537, .F. ) ;
#12532=FACE_OUTER_BOUND ( 'NONE', #22073, .T. ) ;
#12561=ADVANCED_FACE ( 'NONE', ( #17891 ), #3613, .T. ) ;
#12563=ADVANCED_FACE ( 'NONE', ( #1609 ), #21937, .T. ) ;
#12564=DIRECTION ( 'NONE',  ( 0.1000233216789610108, 0.9949850929136109245, -3.588240815588595806E-13 ) ) ;
#12570=CARTESIAN_POINT ( 'NONE',  ( 12.01554901919999985, -37.47280209340000567, -144.5552959529999839 ) ) ;
#12584=ADVANCED_FACE ( 'NONE', ( #16109 ), #1958, .F. ) ;
#12590=DIRECTION ( 'NONE',  ( -0.9892101392001055871, 0.1465035852930155202, 0.000000000000000000 ) ) ;
#12591=EDGE_LOOP ( 'NONE', ( #2051, #10294, #13827, #6443 ) ) ;
#12593=AXIS2_PLACEMENT_3D ( 'NONE', #18709, #18357, #5615 ) ;
#12594=VECTOR ( 'NONE', #13370, 1000.000000000000000 ) ;
#12596=EDGE_CURVE ( 'NONE', #5244, #4587, #8943, .T. ) ;
#12599=DIRECTION ( 'NONE',  ( -0.9919007982877544594, 0.1270149847699686418, 4.766005912188822159E-14 ) ) ;
#12600=EDGE_CURVE ( 'NONE', #12006, #20679, #7664, .T. ) ;
#12627=ORIENTED_EDGE ( 'NONE', *, *, #3909, .T. ) ;
#12631=DIRECTION ( 'NONE',  ( -0.9896415801065049367, 0.1435602414469282218, 8.993136838065500309E-12 ) ) ;
#12644=CARTESIAN_POINT ( 'NONE',  ( 16.61718498210000305, -18.75502267109999721, -142.5552959529999839 ) ) ;
#12645=AXIS2_PLACEMENT_3D ( 'NONE', #1458, #11908, #987 ) ;
#12646=EDGE_LOOP ( 'NONE', ( #13414, #13391, #3496 ) ) ;
#12651=PLANE ( 'NONE',  #12170 ) ;
#12663=DIRECTION ( 'NONE',  ( 1.000000000000000000, 0.000000000000000000, -4.429789868254374596E-12 ) ) ;
#12665=VERTEX_POINT ( 'NONE', #15258 ) ;
#12674=CARTESIAN_POINT ( 'NONE',  ( 2.508811538190000245, -14.35090895149999923, -145.5552959529999839 ) ) ;
#12687=ADVANCED_FACE ( 'NONE', ( #2307 ), #16803, .F. ) ;
#12704=DIRECTION ( 'NONE',  ( -0.9949850929136110356, 0.1000233216789610385, -5.551115123125783491E-15 ) ) ;
#12709=EDGE_CURVE ( 'NONE', #8241, #22607, #13220, .T. ) ;
#12720=DIRECTION ( 'NONE',  ( 1.000000000000000000, 0.000000000000000000, -4.430318231639999944E-12 ) ) ;
#12725=DIRECTION ( 'NONE',  ( -4.430233957459999899E-12, 6.092903959140000514E-13, -1.000000000000000000 ) ) ;
#12732=FACE_OUTER_BOUND ( 'NONE', #11482, .T. ) ;
#12739=ORIENTED_EDGE ( 'NONE', *, *, #12267, .F. ) ;
#12753=ORIENTED_EDGE ( 'NONE', *, *, #6201, .T. ) ;
#12756=PLANE ( 'NONE',  #3503 ) ;
#12757=LINE ( 'NONE', #14205, #8024 ) ;
#12765=CARTESIAN_POINT ( 'NONE',  ( -6.327504759656895850, -17.27997690994742896, -145.5552959530004671 ) ) ;
#12770=DIRECTION ( 'NONE',  ( -0.06298685227120542907, -0.9980143568310855251, 1.534772309240130738E-13 ) ) ;
#12771=CARTESIAN_POINT ( 'NONE',  ( -9.434278515689999978, -18.41834002140000237, -147.5552959529999839 ) ) ;
#12774=PLANE ( 'NONE',  #21889 ) ;
#12775=CARTESIAN_POINT ( 'NONE',  ( 17.44013884619999999, -20.67371738400000325, -144.5552959529999839 ) ) ;
#12776=EDGE_LOOP ( 'NONE', ( #18638, #14531, #23474, #12067 ) ) ;
#12781=ADVANCED_FACE ( 'NONE', ( #4663 ), #5016, .F. ) ;
#12782=ORIENTED_EDGE ( 'NONE', *, *, #8881, .T. ) ;
#12792=LINE ( 'NONE', #14700, #15222 ) ;
#12798=ORIENTED_EDGE ( 'NONE', *, *, #10962, .F. ) ;
#12806=EDGE_LOOP ( 'NONE', ( #3549, #727, #12627, #16729, #22227 ) ) ;
#12807=EDGE_CURVE ( 'NONE', #2580, #361, #11902, .T. ) ;
#12817=CARTESIAN_POINT ( 'NONE',  ( 16.25766103973663945, -22.55971267323774399, -145.5552959530246540 ) ) ;
#12822=ORIENTED_EDGE ( 'NONE', *, *, #4924, .F. ) ;
#12827=VERTEX_POINT ( 'NONE', #1228 ) ;
#12838=EDGE_CURVE ( 'NONE', #12998, #5773, #16413, .T. ) ;
#12844=VECTOR ( 'NONE', #11477, 1000.000000000000000 ) ;
#12848=CARTESIAN_POINT ( 'NONE',  ( 2.068499633510000102, -14.99362786250000035, -148.0552959529999839 ) ) ;
#12849=EDGE_CURVE ( 'NONE', #6393, #712, #1619, .T. ) ;
#12852=EDGE_LOOP ( 'NONE', ( #11290, #9847, #87, #3967, #9563, #5375, #22417 ) ) ;
#12858=EDGE_CURVE ( 'NONE', #4598, #14014, #8025, .T. ) ;
#12872=CARTESIAN_POINT ( 'NONE',  ( -8.916553640509999212, -11.88594259849999979, -143.5552959529999839 ) ) ;
#12874=CARTESIAN_POINT ( 'NONE',  ( 2.508811538200000246, -14.35090895149999923, -144.5552959529999839 ) ) ;
#12887=ADVANCED_FACE ( 'NONE', ( #19773 ), #11283, .F. ) ;
#12897=EDGE_LOOP ( 'NONE', ( #3009, #14276, #4216 ) ) ;
#12909=ORIENTED_EDGE ( 'NONE', *, *, #17667, .T. ) ;
#12912=VECTOR ( 'NONE', #19636, 1000.000000000000227 ) ;
#12913=CIRCLE ( 'NONE', #18631, 15.00000000000000178 ) ;
#12914=EDGE_CURVE ( 'NONE', #2213, #7225, #22488, .T. ) ;
#12930=ORIENTED_EDGE ( 'NONE', *, *, #15852, .T. ) ;
#12933=VECTOR ( 'NONE', #4965, 1000.000000000000000 ) ;
#12938=CARTESIAN_POINT ( 'NONE',  ( -6.547730170590000398, -18.66441632429999942, -148.5552959529999839 ) ) ;
#12946=EDGE_CURVE ( 'NONE', #19545, #8311, #9618, .T. ) ;
#12950=LINE ( 'NONE', #19982, #17350 ) ;
#12953=CARTESIAN_POINT ( 'NONE',  ( 1.357896944619999990, -19.89221232270000073, -148.5552959529999839 ) ) ;
#12959=DIRECTION ( 'NONE',  ( -0.09606172499277226828, -0.9953753789357124848, 8.268133652477615271E-13 ) ) ;
#12962=ORIENTED_EDGE ( 'NONE', *, *, #3555, .F. ) ;
#12965=CARTESIAN_POINT ( 'NONE',  ( 16.29836742280000195, -22.74229684829999698, -143.5552959529999839 ) ) ;
#12983=ORIENTED_EDGE ( 'NONE', *, *, #1401, .F. ) ;
#12996=LINE ( 'NONE', #15372, #22584 ) ;
#12998=VERTEX_POINT ( 'NONE', #20699 ) ;
#13000=VECTOR ( 'NONE', #15442, 1000.000000000000114 ) ;
#13002=ORIENTED_EDGE ( 'NONE', *, *, #13104, .F. ) ;
#13005=ADVANCED_FACE ( 'NONE', ( #2281 ), #9270, .T. ) ;
#13006=DIRECTION ( 'NONE',  ( 2.839308199620000013E-14, 3.568879590630000244E-13, 1.000000000000000000 ) ) ;
#13021=EDGE_LOOP ( 'NONE', ( #12003, #9898, #1082, #7426, #15093 ) ) ;
#13022=ORIENTED_EDGE ( 'NONE', *, *, #1412, .F. ) ;
#13025=CARTESIAN_POINT ( 'NONE',  ( 17.33131581010000133, -22.98361965280000163, -147.0552959529999839 ) ) ;
#13031=CYLINDRICAL_SURFACE ( 'NONE', #5641, 6.000000000000003553 ) ;
#13034=EDGE_CURVE ( 'NONE', #19256, #2929, #2398, .T. ) ;
#13048=ORIENTED_EDGE ( 'NONE', *, *, #13677, .F. ) ;
#13049=CARTESIAN_POINT ( 'NONE',  ( -8.650148125288117384, -11.23751091877166886, -145.5552959530002965 ) ) ;
#13050=EDGE_LOOP ( 'NONE', ( #19222, #7315, #20732, #20309 ) ) ;
#13063=CARTESIAN_POINT ( 'NONE',  ( -7.041959465309999722, -26.08051538799999847, -142.5552959529999839 ) ) ;
#13065=LINE ( 'NONE', #233, #9736 ) ;
#13070=ORIENTED_EDGE ( 'NONE', *, *, #8103, .F. ) ;
#13074=CARTESIAN_POINT ( 'NONE',  ( 16.25412235410000150, -22.59491385829999999, -145.5552959529999839 ) ) ;
#13075=CARTESIAN_POINT ( 'NONE',  ( -0.6781431574009999519, -62.17334590100000469, -147.5552959529999839 ) ) ;
#13079=CARTESIAN_POINT ( 'NONE',  ( 25.15155135439999867, -26.08415009650000016, -147.5552959529999839 ) ) ;
#13080=ADVANCED_FACE ( 'NONE', ( #17480 ), #8428, .T. ) ;
#13084=ADVANCED_FACE ( 'NONE', ( #19391 ), #4747, .F. ) ;
#13090=EDGE_LOOP ( 'NONE', ( #18693, #21581, #21319, #2542, #12072 ) ) ;
#13091=VERTEX_POINT ( 'NONE', #8302 ) ;
#13093=LINE ( 'NONE', #20364, #21907 ) ;
#13097=DIRECTION ( 'NONE',  ( 1.267807176944654053E-15, 0.000000000000000000, 1.000000000000000000 ) ) ;
#13098=CARTESIAN_POINT ( 'NONE',  ( 20.35976161480000002, -31.74228192520000391, -145.5552959529999839 ) ) ;
#13104=EDGE_CURVE ( 'NONE', #3115, #20005, #1203, .T. ) ;
#13106=DIRECTION ( 'NONE',  ( 0.09606172499277226828, 0.9953753789357124848, -8.277822871607614780E-13 ) ) ;
#13108=CARTESIAN_POINT ( 'NONE',  ( 24.36715301250000110, -30.57462384669999977, -147.5552959529999839 ) ) ;
#13111=CARTESIAN_POINT ( 'NONE',  ( 7.200097415480000151, -13.39991276200000136, -144.5552959529999839 ) ) ;
#13113=PRESENTATION_STYLE_ASSIGNMENT (( #5627 ) ) ;
#13119=ORIENTED_EDGE ( 'NONE', *, *, #12946, .F. ) ;
#13122=PLANE ( 'NONE',  #19649 ) ;
#13125=EDGE_CURVE ( 'NONE', #8795, #12291, #19029, .T. ) ;
#13131=ORIENTED_EDGE ( 'NONE', *, *, #20741, .F. ) ;
#13132=AXIS2_PLACEMENT_3D ( 'NONE', #17112, #832, #6278 ) ;
#13135=EDGE_CURVE ( 'NONE', #6792, #2284, #10714, .T. ) ;
#13137=CARTESIAN_POINT ( 'NONE',  ( 5.631397321050000571, -17.85059010000000157, -146.5552959529999839 ) ) ;
#13140=CARTESIAN_POINT ( 'NONE',  ( 12.77456842470000176, -18.14116071520000162, -142.5552959529999839 ) ) ;
#13141=VERTEX_POINT ( 'NONE', #22841 ) ;
#13142=CARTESIAN_POINT ( 'NONE',  ( 1.591914056710000080, -18.48847405160000079, -144.5552959529999839 ) ) ;
#13148=EDGE_LOOP ( 'NONE', ( #19959, #5275, #21354, #16886, #7665, #2400, #14917, #8389, #13922, #4879, #12962, #20798 ) ) ;
#13159=ORIENTED_EDGE ( 'NONE', *, *, #5754, .T. ) ;
#13166=VECTOR ( 'NONE', #17612, 1000.000000000000000 ) ;
#13173=LINE ( 'NONE', #20446, #22777 ) ;
#13178=ADVANCED_FACE ( 'NONE', ( #17126 ), #10080, .F. ) ;
#13184=FACE_OUTER_BOUND ( 'NONE', #3886, .T. ) ;
#13186=DIRECTION ( 'NONE',  ( 1.527666881879999979E-13, 8.153477892850000134E-13, 1.000000000000000000 ) ) ;
#13187=CARTESIAN_POINT ( 'NONE',  ( -8.770737564319999180, -11.35481373070000011, -143.5552959529999839 ) ) ;
#13189=CARTESIAN_POINT ( 'NONE',  ( -8.916553640509999212, -11.88594259849999979, -142.5552959529999839 ) ) ;
#13194=ORIENTED_EDGE ( 'NONE', *, *, #20324, .T. ) ;
#13211=PLANE ( 'NONE',  #14715 ) ;
#13214=DIRECTION ( 'NONE',  ( 9.185449151653098762E-12, 0.000000000000000000, 1.000000000000000000 ) ) ;
#13220=LINE ( 'NONE', #17028, #22117 ) ;
#13223=EDGE_LOOP ( 'NONE', ( #14938, #10374, #12782, #1654, #4511 ) ) ;
#13227=DIRECTION ( 'NONE',  ( -0.07970438983373198671, -0.9968185442904001770, 8.248698894599408818E-13 ) ) ;
#13245=AXIS2_PLACEMENT_3D ( 'NONE', #22943, #19363, #817 ) ;
#13252=ORIENTED_EDGE ( 'NONE', *, *, #5754, .F. ) ;
#13253=VECTOR ( 'NONE', #21803, 1000.000000000000000 ) ;
#13254=CARTESIAN_POINT ( 'NONE',  ( 22.40528270640000130, -21.39206583629999869, -146.5552959529999839 ) ) ;
#13257=LINE ( 'NONE', #13142, #20536 ) ;
#13259=VECTOR ( 'NONE', #4208, 1000.000000000000114 ) ;
#13262=EDGE_CURVE ( 'NONE', #21613, #16855, #16405, .T. ) ;
#13266=PLANE ( 'NONE',  #22851 ) ;
#13272=CARTESIAN_POINT ( 'NONE',  ( -9.395847196590883854, -17.80940328571869102, -146.5552959529997565 ) ) ;
#13273=EDGE_CURVE ( 'NONE', #21143, #16352, #10785, .T. ) ;
#13281=CARTESIAN_POINT ( 'NONE',  ( 1.357896944619999990, -19.89221232270000073, -148.0552959529999839 ) ) ;
#13282=CARTESIAN_POINT ( 'NONE',  ( -0.6781431574009999519, -62.17334590100000469, -147.5552959529999839 ) ) ;
#13284=AXIS2_PLACEMENT_3D ( 'NONE', #9128, #5215, #18072 ) ;
#13286=EDGE_CURVE ( 'NONE', #22422, #6588, #16431, .T. ) ;
#13289=VECTOR ( 'NONE', #846, 1000.000000000000114 ) ;
#13298=CARTESIAN_POINT ( 'NONE',  ( 16.29836742280000195, -22.74229684829999698, -142.5552959529999839 ) ) ;
#13307=CARTESIAN_POINT ( 'NONE',  ( -2.203055323360000095, -15.74846988260000025, -143.5552959529999839 ) ) ;
#13310=EDGE_CURVE ( 'NONE', #10073, #16792, #18184, .T. ) ;
#13321=ADVANCED_FACE ( 'NONE', ( #115 ), #5567, .T. ) ;
#13323=EDGE_CURVE ( 'NONE', #2700, #12291, #1781, .T. ) ;
#13329=DIRECTION ( 'NONE',  ( 1.000000000000000000, 0.000000000000000000, -2.775557561562892298E-14 ) ) ;
#13332=DIRECTION ( 'NONE',  ( 2.839308199605699858E-14, 3.568879590633174872E-13, 1.000000000000000000 ) ) ;
#13337=CARTESIAN_POINT ( 'NONE',  ( -9.347107914279998653, -17.32706600430000066, -143.5552959529999839 ) ) ;
#13357=CARTESIAN_POINT ( 'NONE',  ( 16.61718498210000305, -18.75502267109999721, -143.0552959529999839 ) ) ;
#13364=DIRECTION ( 'NONE',  ( -0.9840552701943220404, 0.1778629393740580045, -3.651917849741195385E-14 ) ) ;
#13370=DIRECTION ( 'NONE',  ( 0.2451800884060535979, 0.9694775522152123681, -1.311492566970288567E-12 ) ) ;
#13371=CIRCLE ( 'NONE', #2004, 5.999999999999998224 ) ;
#13372=AXIS2_PLACEMENT_3D ( 'NONE', #4539, #22628, #6318 ) ;
#13374=EDGE_CURVE ( 'NONE', #361, #10851, #13375, .T. ) ;
#13375=CIRCLE ( 'NONE', #3132, 5.000000000000000000 ) ;
#13378=DIRECTION ( 'NONE',  ( 8.955190032050000935E-12, -9.104778821549999739E-13, 1.000000000000000000 ) ) ;
#13380=EDGE_CURVE ( 'NONE', #30, #21927, #2242, .T. ) ;
#13388=CARTESIAN_POINT ( 'NONE',  ( -6.604791614870066496, -20.14156755886077832, -144.5552959529732959 ) ) ;
#13391=ORIENTED_EDGE ( 'NONE', *, *, #12285, .T. ) ;
#13397=ORIENTED_EDGE ( 'NONE', *, *, #17026, .F. ) ;
#13400=DIRECTION ( 'NONE',  ( 8.955190032050000935E-12, -9.104778821549999739E-13, 1.000000000000000000 ) ) ;
#13402=( GEOMETRIC_REPRESENTATION_CONTEXT ( 3 ) GLOBAL_UNCERTAINTY_ASSIGNED_CONTEXT ( ( #6843 ) ) GLOBAL_UNIT_ASSIGNED_CONTEXT ( ( #16105, #4921, #10135 ) ) REPRESENTATION_CONTEXT ( 'NONE', 'WORKASPACE' ) );
#13407=CARTESIAN_POINT ( 'NONE',  ( -9.347107914279998653, -17.32706600430000066, -143.5552959529999839 ) ) ;
#13409=EDGE_CURVE ( 'NONE', #2618, #1486, #456, .T. ) ;
#13412=DIRECTION ( 'NONE',  ( 0.09606172499277226828, 0.9953753789357124848, -8.277822871607614780E-13 ) ) ;
#13413=PLANE ( 'NONE',  #753 ) ;
#13414=ORIENTED_EDGE ( 'NONE', *, *, #854, .F. ) ;
#13415=CARTESIAN_POINT ( 'NONE',  ( 17.06104532839999877, -32.02344838739999489, -142.5552959529999839 ) ) ;
#13419=ORIENTED_EDGE ( 'NONE', *, *, #12914, .F. ) ;
#13428=VERTEX_POINT ( 'NONE', #7918 ) ;
#13434=VERTEX_POINT ( 'NONE', #12817 ) ;
#13437=ORIENTED_EDGE ( 'NONE', *, *, #7805, .T. ) ;
#13444=CARTESIAN_POINT ( 'NONE',  ( 12.90429904045548426, -17.98118184282727938, -144.5552959530160422 ) ) ;
#13451=CARTESIAN_POINT ( 'NONE',  ( 1.759100530420000030, -16.38142836440000139, -143.5552959529999839 ) ) ;
#13455=CIRCLE ( 'NONE', #10015, 15.00000000000000178 ) ;
#13459=PLANE ( 'NONE',  #13372 ) ;
#13468=CARTESIAN_POINT ( 'NONE',  ( -9.282104535860000283, -16.71402168319999859, -145.5552959529999839 ) ) ;
#13499=LINE ( 'NONE', #15059, #19454 ) ;
#13502=DIRECTION ( 'NONE',  ( -1.527666881879999979E-13, -8.171241461240000022E-13, -1.000000000000000000 ) ) ;
#13507=DIRECTION ( 'NONE',  ( -0.1146332952500066227, -0.9934078757590583120, -9.663381206340560633E-14 ) ) ;
#13508=ORIENTED_EDGE ( 'NONE', *, *, #23330, .F. ) ;
#13521=VECTOR ( 'NONE', #7229, 1000.000000000000114 ) ;
#13532=PLANE ( 'NONE',  #13132 ) ;
#13534=DIRECTION ( 'NONE',  ( 7.389987738588579788E-14, 0.000000000000000000, 1.000000000000000000 ) ) ;
#13546=ORIENTED_EDGE ( 'NONE', *, *, #10626, .F. ) ;
#13547=CARTESIAN_POINT ( 'NONE',  ( -9.282104535849999394, -16.71402168319999859, -144.5552959529999839 ) ) ;
#13549=EDGE_LOOP ( 'NONE', ( #6326, #12229, #6643 ) ) ;
#13559=DIRECTION ( 'NONE',  ( -8.955503005839999404E-12, 9.094947017729999296E-13, -1.000000000000000000 ) ) ;
#13566=ORIENTED_EDGE ( 'NONE', *, *, #3278, .F. ) ;
#13568=CIRCLE ( 'NONE', #1828, 15.00000000000000178 ) ;
#13570=ADVANCED_FACE ( 'NONE', ( #12207 ), #3402, .T. ) ;
#13576=DIRECTION ( 'NONE',  ( -1.526468026909999897E-13, -8.159623473500000156E-13, -1.000000000000000000 ) ) ;
#13578=FACE_OUTER_BOUND ( 'NONE', #19155, .T. ) ;
#13582=ADVANCED_FACE ( 'NONE', ( #17686 ), #16260, .F. ) ;
#13604=DIRECTION ( 'NONE',  ( 1.000000000000000000, 0.000000000000000000, -8.953948693601887499E-12 ) ) ;
#13605=VECTOR ( 'NONE', #11636, 1000.000000000000227 ) ;
#13606=EDGE_LOOP ( 'NONE', ( #23040, #15984, #12983 ) ) ;
#13608=PLANE ( 'NONE',  #6076 ) ;
#13609=CIRCLE ( 'NONE', #15903, 5.999999999999998224 ) ;
#13610=ORIENTED_EDGE ( 'NONE', *, *, #13286, .F. ) ;
#13614=EDGE_CURVE ( 'NONE', #4947, #22537, #4672, .T. ) ;
#13620=AXIS2_PLACEMENT_3D ( 'NONE', #17581, #8518, #4843 ) ;
#13625=ORIENTED_EDGE ( 'NONE', *, *, #13867, .T. ) ;
#13629=DIRECTION ( 'NONE',  ( 1.000000000000000000, 0.000000000000000000, -2.775557561562891351E-14 ) ) ;
#13630=VERTEX_POINT ( 'NONE', #16920 ) ;
#13637=DIRECTION ( 'NONE',  ( -0.1146332952500066227, -0.9934078757590583120, -9.663381206340560633E-14 ) ) ;
#13643=AXIS2_PLACEMENT_3D ( 'NONE', #4357, #8393, #13629 ) ;
#13653=ORIENTED_EDGE ( 'NONE', *, *, #1484, .T. ) ;
#13656=VERTEX_POINT ( 'NONE', #7866 ) ;
#13659=ORIENTED_EDGE ( 'NONE', *, *, #2438, .T. ) ;
#13663=VERTEX_POINT ( 'NONE', #7985 ) ;
#13665=VECTOR ( 'NONE', #6262, 999.9999999999998863 ) ;
#13667=ORIENTED_EDGE ( 'NONE', *, *, #13374, .F. ) ;
#13670=DIRECTION ( 'NONE',  ( 8.740345284041279692E-14, 0.000000000000000000, 1.000000000000000000 ) ) ;
#13671=ORIENTED_EDGE ( 'NONE', *, *, #2044, .T. ) ;
#13672=DIRECTION ( 'NONE',  ( 1.000000000000000000, 0.000000000000000000, -4.511206223393553012E-12 ) ) ;
#13673=EDGE_LOOP ( 'NONE', ( #4119, #5493, #15218, #9322, #16346, #19582 ) ) ;
#13677=EDGE_CURVE ( 'NONE', #22537, #320, #6177, .T. ) ;
#13680=ORIENTED_EDGE ( 'NONE', *, *, #16949, .F. ) ;
#13682=VECTOR ( 'NONE', #7433, 1000.000000000000114 ) ;
#13683=DIRECTION ( 'NONE',  ( 8.955190032050000935E-12, -9.104778821549999739E-13, 1.000000000000000000 ) ) ;
#13686=DIRECTION ( 'NONE',  ( 1.000000000000000000, 0.000000000000000000, -4.429789868254373788E-12 ) ) ;
#13688=ORIENTED_EDGE ( 'NONE', *, *, #20975, .F. ) ;
#13692=DIRECTION ( 'NONE',  ( -4.430233957459999899E-12, 6.110667527539999876E-13, -1.000000000000000000 ) ) ;
#13693=CARTESIAN_POINT ( 'NONE',  ( 23.78818517497825269, -17.51387386319285611, -142.5552959530024566 ) ) ;
#13698=DIRECTION ( 'NONE',  ( 1.000000000000000000, 0.000000000000000000, -2.854859206178974232E-14 ) ) ;
#13716=EDGE_CURVE ( 'NONE', #2388, #22098, #11663, .T. ) ;
#13728=ORIENTED_EDGE ( 'NONE', *, *, #5491, .F. ) ;
#13734=EDGE_LOOP ( 'NONE', ( #1682, #10842, #189, #3971, #12462, #3501 ) ) ;
#13736=LINE ( 'NONE', #18130, #2672 ) ;
#13738=EDGE_CURVE ( 'NONE', #13428, #10483, #20255, .T. ) ;
#13739=ORIENTED_EDGE ( 'NONE', *, *, #936, .T. ) ;
#13746=EDGE_CURVE ( 'NONE', #10483, #14227, #15375, .T. ) ;
#13752=DIRECTION ( 'NONE',  ( 0.000000000000000000, -1.000000000000000000, 8.159623473500000156E-13 ) ) ;
#13753=VECTOR ( 'NONE', #9371, 1000.000000000000000 ) ;
#13756=AXIS2_PLACEMENT_3D ( 'NONE', #6789, #6557, #19171 ) ;
#13759=ADVANCED_FACE ( 'NONE', ( #10466 ), #22744, .T. ) ;
#13763=ORIENTED_EDGE ( 'NONE', *, *, #16266, .T. ) ;
#13766=EDGE_CURVE ( 'NONE', #18172, #10602, #14061, .T. ) ;
#13769=ADVANCED_FACE ( 'NONE', ( #10240 ), #15486, .T. ) ;
#13773=DIRECTION ( 'NONE',  ( 8.952838470580000762E-12, -9.094947017729999296E-13, 1.000000000000000000 ) ) ;
#13775=ORIENTED_EDGE ( 'NONE', *, *, #14469, .T. ) ;
#13795=ORIENTED_EDGE ( 'NONE', *, *, #7673, .T. ) ;
#13803=ORIENTED_EDGE ( 'NONE', *, *, #2136, .T. ) ;
#13813=ORIENTED_EDGE ( 'NONE', *, *, #2127, .T. ) ;
#13815=DIRECTION ( 'NONE',  ( -0.1309625047069831461, -0.9913873220698726785, 3.575326271489538320E-13 ) ) ;
#13827=ORIENTED_EDGE ( 'NONE', *, *, #19537, .T. ) ;
#13829=DIRECTION ( 'NONE',  ( 0.9999976651796518290, -0.002160933882609249439, -8.955304954746877373E-12 ) ) ;
#13848=ORIENTED_EDGE ( 'NONE', *, *, #3842, .F. ) ;
#13852=ORIENTED_EDGE ( 'NONE', *, *, #1543, .T. ) ;
#13853=CARTESIAN_POINT ( 'NONE',  ( 2.508811538200000246, -14.35090895149999923, -144.5552959529999839 ) ) ;
#13855=ORIENTED_EDGE ( 'NONE', *, *, #3740, .F. ) ;
#13867=EDGE_CURVE ( 'NONE', #15451, #21143, #22876, .T. ) ;
#13869=ORIENTED_EDGE ( 'NONE', *, *, #13262, .F. ) ;
#13871=VECTOR ( 'NONE', #18455, 1000.000000000000000 ) ;
#13884=FACE_OUTER_BOUND ( 'NONE', #12322, .T. ) ;
#13887=ADVANCED_FACE ( 'NONE', ( #12146 ), #17632, .T. ) ;
#13904=EDGE_LOOP ( 'NONE', ( #3655, #22208, #22256, #1812, #15823 ) ) ;
#13906=VECTOR ( 'NONE', #3689, 1000.000000000000000 ) ;
#13909=AXIS2_PLACEMENT_3D ( 'NONE', #17997, #5381, #20138 ) ;
#13914=EDGE_CURVE ( 'NONE', #12665, #22329, #8808, .T. ) ;
#13915=EDGE_CURVE ( 'NONE', #2213, #12155, #28, .T. ) ;
#13916=ORIENTED_EDGE ( 'NONE', *, *, #16490, .F. ) ;
#13922=ORIENTED_EDGE ( 'NONE', *, *, #5957, .F. ) ;
#13925=CARTESIAN_POINT ( 'NONE',  ( -9.334216945200001447, -17.19633444960000190, -146.5552959529999839 ) ) ;
#13926=LINE ( 'NONE', #2991, #10613 ) ;
#13928=CARTESIAN_POINT ( 'NONE',  ( 22.42370904790000097, -21.41421288319999761, -142.5552959529999839 ) ) ;
#13929=ORIENTED_EDGE ( 'NONE', *, *, #18117, .F. ) ;
#13931=CARTESIAN_POINT ( 'NONE',  ( -6.370493725010000219, -17.65251768590000125, -144.5552959529999839 ) ) ;
#13936=FACE_OUTER_BOUND ( 'NONE', #13148, .T. ) ;
#13954=PLANE ( 'NONE',  #19810 ) ;
#13955=ORIENTED_EDGE ( 'NONE', *, *, #15313, .T. ) ;
#13958=PRESENTATION_STYLE_ASSIGNMENT (( #23009 ) ) ;
#13960=ORIENTED_EDGE ( 'NONE', *, *, #14904, .T. ) ;
#13966=DIRECTION ( 'NONE',  ( 1.000000000000000000, 0.000000000000000000, -4.511206223393553012E-12 ) ) ;
#13973=EDGE_CURVE ( 'NONE', #16462, #13434, #18221, .T. ) ;
#13975=DIRECTION ( 'NONE',  ( -4.511946372079999833E-12, 1.314504061159999897E-13, -1.000000000000000000 ) ) ;
#13976=DIRECTION ( 'NONE',  ( 1.000000000000000000, 0.000000000000000000, -4.510281037539699253E-12 ) ) ;
#13981=VECTOR ( 'NONE', #4305, 1000.000000000000000 ) ;
#13982=ORIENTED_EDGE ( 'NONE', *, *, #16214, .F. ) ;
#13995=ORIENTED_EDGE ( 'NONE', *, *, #5801, .T. ) ;
#13997=EDGE_CURVE ( 'NONE', #21066, #16352, #3825, .T. ) ;
#14002=CARTESIAN_POINT ( 'NONE',  ( 16.61718498210000305, -18.75502267109999721, -142.5552959529999839 ) ) ;
#14005=AXIS2_PLACEMENT_3D ( 'NONE', #7246, #16516, #12590 ) ;
#14010=CARTESIAN_POINT ( 'NONE',  ( 15.85402906740000084, -26.57485422999999969, -145.5552959529999839 ) ) ;
#14011=ORIENTED_EDGE ( 'NONE', *, *, #11404, .T. ) ;
#14013=CARTESIAN_POINT ( 'NONE',  ( 15.59498359470000040, -26.23371093219999750, -147.5552959529999839 ) ) ;
#14014=VERTEX_POINT ( 'NONE', #16439 ) ;
#14025=ORIENTED_EDGE ( 'NONE', *, *, #16069, .T. ) ;
#14026=CARTESIAN_POINT ( 'NONE',  ( 5.631397321050000571, -17.85059010000000157, -147.5552959529999839 ) ) ;
#14032=VERTEX_POINT ( 'NONE', #21563 ) ;
#14036=EDGE_CURVE ( 'NONE', #8980, #13091, #3470, .T. ) ;
#14037=AXIS2_PLACEMENT_3D ( 'NONE', #2865, #6424, #6306 ) ;
#14047=CARTESIAN_POINT ( 'NONE',  ( 1.847645635000000119, -15.93876195360000025, -145.5552959529999839 ) ) ;
#14058=DIRECTION ( 'NONE',  ( -0.9847555042252370550, 0.1739442350240419932, 7.303835699471759765E-15 ) ) ;
#14061=LINE ( 'NONE', #10118, #5438 ) ;
#14065=CIRCLE ( 'NONE', #2673, 35.00000000000000000 ) ;
#14081=AXIS2_PLACEMENT_3D ( 'NONE', #1686, #16186, #23441 ) ;
#14085=EDGE_CURVE ( 'NONE', #320, #18387, #12094, .T. ) ;
#14091=CARTESIAN_POINT ( 'NONE',  ( 16.74346552629999962, -18.31657829129999726, -147.5552959529999839 ) ) ;
#14094=CARTESIAN_POINT ( 'NONE',  ( 16.74346552629999962, -18.31657829129999726, -147.5552959529999839 ) ) ;
#14100=CARTESIAN_POINT ( 'NONE',  ( 23.89222110089999873, -31.59487100459999809, -146.5552959529999839 ) ) ;
#14102=PLANE ( 'NONE',  #8219 ) ;
#14103=LINE ( 'NONE', #23381, #19236 ) ;
#14119=DIRECTION ( 'NONE',  ( 4.430318231639999944E-12, -6.100259101500000139E-13, 1.000000000000000000 ) ) ;
#14122=CARTESIAN_POINT ( 'NONE',  ( -6.363831972638722689, -17.39670249660616363, -147.5552959530002681 ) ) ;
#14129=VECTOR ( 'NONE', #8449, 1000.000000000000000 ) ;
#14131=AXIS2_PLACEMENT_3D ( 'NONE', #21587, #5509, #3726 ) ;
#14132=VECTOR ( 'NONE', #11405, 999.9999999999998863 ) ;
#14135=DIRECTION ( 'NONE',  ( -1.843274626514380137E-11, 0.000000000000000000, -1.000000000000000000 ) ) ;
#14141=EDGE_CURVE ( 'NONE', #21927, #17682, #7182, .T. ) ;
#14152=DIRECTION ( 'NONE',  ( 1.000000000000000000, 0.000000000000000000, -2.715621035259064790E-14 ) ) ;
#14153=VECTOR ( 'NONE', #14880, 1000.000000000000114 ) ;
#14159=ADVANCED_FACE ( 'NONE', ( #15109, #5947, #15237 ), #20359, .T. ) ;
#14163=EDGE_LOOP ( 'NONE', ( #3993, #9242, #13955, #808 ) ) ;
#14164=CARTESIAN_POINT ( 'NONE',  ( 22.27792782919999937, -15.32580087659999890, -145.0552959529999839 ) ) ;
#14165=FACE_OUTER_BOUND ( 'NONE', #14818, .T. ) ;
#14174=CARTESIAN_POINT ( 'NONE',  ( -9.317785202249279308, -17.02322901197889848, -144.5552959530000123 ) ) ;
#14177=CARTESIAN_POINT ( 'NONE',  ( 2.531727043930000143, -11.80034048859999807, -147.5552959529999839 ) ) ;
#14187=DIRECTION ( 'NONE',  ( 1.000000000000000000, 0.000000000000000000, -4.510281037539699253E-12 ) ) ;
#14205=CARTESIAN_POINT ( 'NONE',  ( -6.603585321229999749, -20.59801339440000234, -142.5552959529999839 ) ) ;
#14209=CARTESIAN_POINT ( 'NONE',  ( 17.44013884619999999, -20.67371738400000325, -145.5552959529999839 ) ) ;
#14215=PLANE ( 'NONE',  #2508 ) ;
#14217=EDGE_CURVE ( 'NONE', #5894, #9011, #1206, .T. ) ;
#14227=VERTEX_POINT ( 'NONE', #22847 ) ;
#14232=ORIENTED_EDGE ( 'NONE', *, *, #20447, .T. ) ;
#14235=VECTOR ( 'NONE', #16436, 1000.000000000000227 ) ;
#14244=EDGE_CURVE ( 'NONE', #5226, #1779, #17608, .T. ) ;
#14247=EDGE_LOOP ( 'NONE', ( #13995, #698, #10067, #9778, #15170 ) ) ;
#14265=DIRECTION ( 'NONE',  ( -0.9753087663813413410, 0.2208456705930775810, 8.936242978303132921E-12 ) ) ;
#14269=EDGE_CURVE ( 'NONE', #17671, #11516, #21183, .T. ) ;
#14272=CARTESIAN_POINT ( 'NONE',  ( -2.203055323360000095, -15.74846988260000025, -143.5552959529999839 ) ) ;
#14276=ORIENTED_EDGE ( 'NONE', *, *, #9433, .F. ) ;
#14279=CARTESIAN_POINT ( 'NONE',  ( -9.282104535860000283, -16.71402168319999859, -145.5552959529999839 ) ) ;
#14290=DIRECTION ( 'NONE',  ( 0.000000000000000000, -1.000000000000000000, 3.568879590630000244E-13 ) ) ;
#14294=CARTESIAN_POINT ( 'NONE',  ( -9.157754307290000284, -15.75963164970000108, -147.5552959529999839 ) ) ;
#14298=CARTESIAN_POINT ( 'NONE',  ( -2.121568318600000058, -15.32705806070000243, -144.5552959529999839 ) ) ;
#14299=ORIENTED_EDGE ( 'NONE', *, *, #23215, .T. ) ;
#14310=ORIENTED_EDGE ( 'NONE', *, *, #50, .F. ) ;
#14319=PLANE ( 'NONE',  #10629 ) ;
#14320=LINE ( 'NONE', #3618, #7961 ) ;
#14328=DIRECTION ( 'NONE',  ( -4.510774274160000731E-12, 1.321907670990000086E-13, -1.000000000000000000 ) ) ;
#14330=CARTESIAN_POINT ( 'NONE',  ( -9.434278515689999978, -18.41834002140000237, -147.5552959529999839 ) ) ;
#14343=CARTESIAN_POINT ( 'NONE',  ( -6.601136089949999786, -20.10368962670000315, -143.5552959529999839 ) ) ;
#14349=ADVANCED_FACE ( 'NONE', ( #3095 ), #5216, .T. ) ;
#14352=DIRECTION ( 'NONE',  ( 4.569805223421110083E-12, 0.000000000000000000, 1.000000000000000000 ) ) ;
#14353=ORIENTED_EDGE ( 'NONE', *, *, #23188, .T. ) ;
#14354=CARTESIAN_POINT ( 'NONE',  ( 5.631397321050000571, -17.85059010000000157, -147.5552959529999839 ) ) ;
#14356=APPLICATION_CONTEXT ( 'automotive_design' ) ;
#14359=CARTESIAN_POINT ( 'NONE',  ( -6.657076963140000636, -20.13603737529999904, -145.0552959529999839 ) ) ;
#14363=CARTESIAN_POINT ( 'NONE',  ( 2.016283561950000358, -13.16498300129999954, -142.5552959529999839 ) ) ;
#14365=VERTEX_POINT ( 'NONE', #3318 ) ;
#14376=ORIENTED_EDGE ( 'NONE', *, *, #21351, .F. ) ;
#14379=CARTESIAN_POINT ( 'NONE',  ( 2.531727043930000143, -11.80034048859999807, -147.5552959529999839 ) ) ;
#14386=AXIS2_PLACEMENT_3D ( 'NONE', #12570, #21280, #8758 ) ;
#14388=ORIENTED_EDGE ( 'NONE', *, *, #1675, .F. ) ;
#14390=CARTESIAN_POINT ( 'NONE',  ( -9.334216945200001447, -17.19633444960000190, -145.5552959529999839 ) ) ;
#14394=CARTESIAN_POINT ( 'NONE',  ( 16.07620488043449569, -22.91638164385598841, -147.5552959530484429 ) ) ;
#14403=ADVANCED_FACE ( 'NONE', ( #8478 ), #9248, .T. ) ;
#14405=VECTOR ( 'NONE', #9849, 999.9999999999998863 ) ;
#14406=CARTESIAN_POINT ( 'NONE',  ( 15.59498359470000040, -26.23371093219999750, -148.5552959529999839 ) ) ;
#14415=FACE_OUTER_BOUND ( 'NONE', #6529, .T. ) ;
#14420=VECTOR ( 'NONE', #6263, 1000.000000000000114 ) ;
#14427=ORIENTED_EDGE ( 'NONE', *, *, #7168, .F. ) ;
#14432=ORIENTED_EDGE ( 'NONE', *, *, #18801, .T. ) ;
#14435=DIRECTION ( 'NONE',  ( -0.9892101392001054760, 0.1465035852930155480, 4.471739159800472250E-12 ) ) ;
#14436=LINE ( 'NONE', #20496, #463 ) ;
#14440=VECTOR ( 'NONE', #5400, 999.9999999999998863 ) ;
#14452=CARTESIAN_POINT ( 'NONE',  ( -8.594304764359998572, -10.75357442870000035, -145.5552959529999839 ) ) ;
#14454=DIRECTION ( 'NONE',  ( 4.430318231639999944E-12, -6.100259101500000139E-13, 1.000000000000000000 ) ) ;
#14456=CARTESIAN_POINT ( 'NONE',  ( 17.33131581010000133, -22.98361965280000163, -146.5552959529999839 ) ) ;
#14469=EDGE_CURVE ( 'NONE', #11485, #6588, #5571, .T. ) ;
#14470=DIRECTION ( 'NONE',  ( -0.1000233216789610108, -0.9949850929136109245, 3.559993607998610461E-13 ) ) ;
#14471=ORIENTED_EDGE ( 'NONE', *, *, #13973, .F. ) ;
#14476=AXIS2_PLACEMENT_3D ( 'NONE', #14279, #7136, #12720 ) ;
#14481=EDGE_CURVE ( 'NONE', #14876, #15664, #15148, .T. ) ;
#14485=DIRECTION ( 'NONE',  ( -1.527666881879999979E-13, -8.171241461240000022E-13, -1.000000000000000000 ) ) ;
#14488=ADVANCED_FACE ( 'NONE', ( #14619 ), #21886, .F. ) ;
#14490=ORIENTED_EDGE ( 'NONE', *, *, #3446, .F. ) ;
#14494=AXIS2_PLACEMENT_3D ( 'NONE', #5975, #7641, #13227 ) ;
#14505=CARTESIAN_POINT ( 'NONE',  ( -1.844824604560000081, -14.10750774809999974, -147.5552959529999839 ) ) ;
#14506=DIRECTION ( 'NONE',  ( 4.430318231639999944E-12, -6.100259101500000139E-13, 1.000000000000000000 ) ) ;
#14507=ORIENTED_EDGE ( 'NONE', *, *, #10463, .F. ) ;
#14510=DIRECTION ( 'NONE',  ( 1.526468026909999897E-13, 8.159623473500000156E-13, 1.000000000000000000 ) ) ;
#14516=FACE_OUTER_BOUND ( 'NONE', #8824, .T. ) ;
#14524=LINE ( 'NONE', #14164, #10535 ) ;
#14531=ORIENTED_EDGE ( 'NONE', *, *, #6259, .F. ) ;
#14544=CARTESIAN_POINT ( 'NONE',  ( -6.049191701419999845, -14.51144913589999952, -145.5552959529999839 ) ) ;
#14546=VECTOR ( 'NONE', #17714, 999.9999999999998863 ) ;
#14552=ORIENTED_EDGE ( 'NONE', *, *, #21704, .T. ) ;
#14555=CARTESIAN_POINT ( 'NONE',  ( -2.121568318600000058, -15.32705806070000243, -143.5552959529999839 ) ) ;
#14560=EDGE_LOOP ( 'NONE', ( #1040, #15937, #21575, #16685, #17175 ) ) ;
#14561=FACE_OUTER_BOUND ( 'NONE', #11911, .T. ) ;
#14562=PLANE ( 'NONE',  #14131 ) ;
#14563=PLANE ( 'NONE',  #7746 ) ;
#14569=CARTESIAN_POINT ( 'NONE',  ( 16.87269471589999981, -31.91616505980000085, -143.5552959529999839 ) ) ;
#14577=EDGE_CURVE ( 'NONE', #16847, #19447, #7465, .T. ) ;
#14579=DIRECTION ( 'NONE',  ( 1.526468026909999897E-13, 8.159623473500000156E-13, 1.000000000000000000 ) ) ;
#14580=ORIENTED_EDGE ( 'NONE', *, *, #1503, .F. ) ;
#14582=ORIENTED_EDGE ( 'NONE', *, *, #1484, .F. ) ;
#14586=LINE ( 'NONE', #3526, #20286 ) ;
#14590=DIRECTION ( 'NONE',  ( -0.1000233216789610108, -0.9949850929136109245, 3.600083194518594546E-13 ) ) ;
#14592=DIRECTION ( 'NONE',  ( -1.527666881879999979E-13, -8.171241461240000022E-13, -1.000000000000000000 ) ) ;
#14594=ORIENTED_EDGE ( 'NONE', *, *, #18120, .F. ) ;
#14598=EDGE_CURVE ( 'NONE', #11995, #23456, #19119, .T. ) ;
#14603=LINE ( 'NONE', #5556, #6698 ) ;
#14604=VERTEX_POINT ( 'NONE', #22817 ) ;
#14610=ORIENTED_EDGE ( 'NONE', *, *, #15638, .F. ) ;
#14619=FACE_OUTER_BOUND ( 'NONE', #10359, .T. ) ;
#14628=LINE ( 'NONE', #21663, #5519 ) ;
#14643=FACE_OUTER_BOUND ( 'NONE', #2427, .T. ) ;
#14648=DIRECTION ( 'NONE',  ( 0.1000233216789610108, 0.9949850929136109245, -3.588240815588595806E-13 ) ) ;
#14650=CARTESIAN_POINT ( 'NONE',  ( -9.923478264230000789, -23.29931827799999766, -143.5552959529999839 ) ) ;
#14664=CARTESIAN_POINT ( 'NONE',  ( 22.36721601470000209, -21.34320095609999868, -147.5552959529999839 ) ) ;
#14668=CARTESIAN_POINT ( 'NONE',  ( 12.91075631260000023, -38.04527125359999928, -147.5552959529999839 ) ) ;
#14669=VERTEX_POINT ( 'NONE', #22538 ) ;
#14676=( NAMED_UNIT ( * ) SI_UNIT ( $, .STERADIAN. ) SOLID_ANGLE_UNIT ( ) );
#14677=DIRECTION ( 'NONE',  ( 0.000000000000000000, 7.159923868353169372E-11, -1.000000000000000000 ) ) ;
#14678=CARTESIAN_POINT ( 'NONE',  ( 20.58976242830000203, -31.80400447969999789, -142.5552959529999839 ) ) ;
#14680=DIRECTION ( 'NONE',  ( -1.527666881879999979E-13, -8.171241461240000022E-13, -1.000000000000000000 ) ) ;
#14681=DIRECTION ( 'NONE',  ( 1.000000000000000000, 0.000000000000000000, -4.510774274160000731E-12 ) ) ;
#14682=DIRECTION ( 'NONE',  ( -0.1000233216789610108, -0.9949850929136109245, 3.600083194518594546E-13 ) ) ;
#14688=ORIENTED_EDGE ( 'NONE', *, *, #3995, .T. ) ;
#14690=DIRECTION ( 'NONE',  ( 4.430318231636154847E-12, -6.100259101445539707E-13, 1.000000000000000000 ) ) ;
#14691=CARTESIAN_POINT ( 'NONE',  ( -9.394779979509999990, -17.86685386420000299, -143.5552959529999839 ) ) ;
#14694=EDGE_CURVE ( 'NONE', #15850, #2337, #6805, .T. ) ;
#14695=CARTESIAN_POINT ( 'NONE',  ( 1.829659965300000080, -16.02499107890000118, -144.5552959529999839 ) ) ;
#14700=CARTESIAN_POINT ( 'NONE',  ( 8.931951867280000457, -17.52729875919999714, -143.0552959529999839 ) ) ;
#14715=AXIS2_PLACEMENT_3D ( 'NONE', #735, #7972, #13097 ) ;
#14718=ORIENTED_EDGE ( 'NONE', *, *, #13125, .T. ) ;
#14731=VECTOR ( 'NONE', #13692, 1000.000000000000000 ) ;
#14736=DIRECTION ( 'NONE',  ( 0.9944529286486341046, -0.1051825684329612265, -4.470295960598355531E-12 ) ) ;
#14744=CARTESIAN_POINT ( 'NONE',  ( 23.21181482502168336, -23.48612613680713679, -144.7152959529975362 ) ) ;
#14752=VECTOR ( 'NONE', #5758, 1000.000000000000227 ) ;
#14753=LINE ( 'NONE', #12965, #3068 ) ;
#14754=DIRECTION ( 'NONE',  ( 1.526468026909680062E-13, 8.159623473499330697E-13, 1.000000000000000000 ) ) ;
#14755=CIRCLE ( 'NONE', #14386, 9.999999999999998224 ) ;
#14776=VECTOR ( 'NONE', #12228, 1000.000000000000000 ) ;
#14782=ADVANCED_FACE ( 'NONE', ( #7586 ), #20225, .F. ) ;
#14789=VECTOR ( 'NONE', #20676, 999.9999999999998863 ) ;
#14794=VERTEX_POINT ( 'NONE', #578 ) ;
#14795=CARTESIAN_POINT ( 'NONE',  ( 17.21087225569999646, -22.66053313549999970, -145.5552959529999839 ) ) ;
#14796=VECTOR ( 'NONE', #12231, 1000.000000000000114 ) ;
#14799=CARTESIAN_POINT ( 'NONE',  ( 2.170391987449999505, -12.72823260819999902, -146.5552959529999839 ) ) ;
#14813=VECTOR ( 'NONE', #3908, 1000.000000000000000 ) ;
#14814=AXIS2_PLACEMENT_3D ( 'NONE', #6376, #17683, #11842 ) ;
#14818=EDGE_LOOP ( 'NONE', ( #6822, #16998, #12459, #6859, #13916, #13869 ) ) ;
#14834=EDGE_CURVE ( 'NONE', #6817, #23414, #18195, .T. ) ;
#14838=EDGE_CURVE ( 'NONE', #15850, #19030, #1912, .T. ) ;
#14845=ORIENTED_EDGE ( 'NONE', *, *, #19723, .F. ) ;
#14853=DIRECTION ( 'NONE',  ( 0.000000000000000000, -1.000000000000000000, 3.568879590630000244E-13 ) ) ;
#14855=DIRECTION ( 'NONE',  ( 8.956391184260000029E-12, -9.094947017729999296E-13, 1.000000000000000000 ) ) ;
#14866=CYLINDRICAL_SURFACE ( 'NONE', #7945, 5.000000000000001776 ) ;
#14876=VERTEX_POINT ( 'NONE', #7701 ) ;
#14878=DIRECTION ( 'NONE',  ( -0.1000233216789610108, -0.9949850929136109245, 3.591470555298595137E-13 ) ) ;
#14880=DIRECTION ( 'NONE',  ( 0.9834926989016489207, 0.1809478134909354718, -4.411697319228424767E-12 ) ) ;
#14882=AXIS2_PLACEMENT_3D ( 'NONE', #5482, #10700, #10929 ) ;
#14889=CYLINDRICAL_SURFACE ( 'NONE', #16957, 8.176568160359995119 ) ;
#14894=CARTESIAN_POINT ( 'NONE',  ( 22.01137100460000084, -15.39610142400000115, -147.0552959529999839 ) ) ;
#14895=ADVANCED_FACE ( 'NONE', ( #14516 ), #10913, .T. ) ;
#14904=EDGE_CURVE ( 'NONE', #7225, #30, #13173, .T. ) ;
#14916=DIRECTION ( 'NONE',  ( 1.000000000000000000, 0.000000000000000000, -1.522591576628786004E-13 ) ) ;
#14917=ORIENTED_EDGE ( 'NONE', *, *, #2724, .T. ) ;
#14924=CARTESIAN_POINT ( 'NONE',  ( 7.085709294149999060, -13.66851965709999916, -143.5552959529999839 ) ) ;
#14929=ORIENTED_EDGE ( 'NONE', *, *, #18339, .T. ) ;
#14932=DIRECTION ( 'NONE',  ( 1.000000000000000000, 0.000000000000000000, -1.526556658859589738E-13 ) ) ;
#14933=ADVANCED_FACE ( 'NONE', ( #22821 ), #22581, .F. ) ;
#14938=ORIENTED_EDGE ( 'NONE', *, *, #6605, .F. ) ;
#14948=ORIENTED_EDGE ( 'NONE', *, *, #12914, .T. ) ;
#14956=ORIENTED_EDGE ( 'NONE', *, *, #18336, .F. ) ;
#14958=ORIENTED_EDGE ( 'NONE', *, *, #13716, .F. ) ;
#14967=LINE ( 'NONE', #13407, #14789 ) ;
#14970=VERTEX_POINT ( 'NONE', #6039 ) ;
#14977=LINE ( 'NONE', #2261, #7512 ) ;
#14980=PLANE ( 'NONE',  #3414 ) ;
#14981=LINE ( 'NONE', #4277, #4638 ) ;
#14983=PLANE ( 'NONE',  #15142 ) ;
#14988=EDGE_LOOP ( 'NONE', ( #23465, #16619, #4249, #9333 ) ) ;
#14991=CYLINDRICAL_SURFACE ( 'NONE', #22037, 6.000000000000004441 ) ;
#14996=LINE ( 'NONE', #4293, #7898 ) ;
#14998=ORIENTED_EDGE ( 'NONE', *, *, #6605, .T. ) ;
#15002=FACE_OUTER_BOUND ( 'NONE', #1652, .T. ) ;
#15006=LINE ( 'NONE', #11769, #17694 ) ;
#15008=DIRECTION ( 'NONE',  ( 4.510774274160000731E-12, -1.321907670990000086E-13, 1.000000000000000000 ) ) ;
#15014=DIRECTION ( 'NONE',  ( 0.000000000000000000, -7.444689577964079813E-14, -1.000000000000000000 ) ) ;
#15029=DIRECTION ( 'NONE',  ( 0.000000000000000000, 7.657380550038349542E-13, -1.000000000000000000 ) ) ;
#15033=ORIENTED_EDGE ( 'NONE', *, *, #9279, .F. ) ;
#15041=CARTESIAN_POINT ( 'NONE',  ( 23.99773978629999860, -29.25880395889999974, -148.5552959529999839 ) ) ;
#15047=EDGE_CURVE ( 'NONE', #8241, #19376, #3413, .T. ) ;
#15059=CARTESIAN_POINT ( 'NONE',  ( 24.41610067590000099, -29.22497285029999858, -144.5552959529999839 ) ) ;
#15068=ORIENTED_EDGE ( 'NONE', *, *, #7473, .F. ) ;
#15093=ORIENTED_EDGE ( 'NONE', *, *, #9897, .F. ) ;
#15104=FACE_BOUND ( 'NONE', #16836, .T. ) ;
#15109=FACE_BOUND ( 'NONE', #17110, .T. ) ;
#15113=VERTEX_POINT ( 'NONE', #20196 ) ;
#15115=CARTESIAN_POINT ( 'NONE',  ( 22.40528270640000130, -21.39206583629999869, -145.5552959529999839 ) ) ;
#15117=CARTESIAN_POINT ( 'NONE',  ( 17.66940543669999997, -18.68690163239999791, -144.5552959529999839 ) ) ;
#15133=CARTESIAN_POINT ( 'NONE',  ( 4.374398326270000581, -26.09174856970000178, -143.5552959529999839 ) ) ;
#15134=DIRECTION ( 'NONE',  ( -0.1146332952500066227, -0.9934078757590583120, -1.023181539490060155E-13 ) ) ;
#15142=AXIS2_PLACEMENT_3D ( 'NONE', #22478, #2499, #22243 ) ;
#15147=DIRECTION ( 'NONE',  ( -0.1435602414469281940, -0.9896415801065048257, 3.849849731938073961E-13 ) ) ;
#15148=CIRCLE ( 'NONE', #7909, 8.176568160360000448 ) ;
#15160=ORIENTED_EDGE ( 'NONE', *, *, #20971, .T. ) ;
#15164=CIRCLE ( 'NONE', #3772, 35.00000000000000000 ) ;
#15165=ORIENTED_EDGE ( 'NONE', *, *, #1065, .F. ) ;
#15170=ORIENTED_EDGE ( 'NONE', *, *, #11263, .F. ) ;
#15174=CIRCLE ( 'NONE', #17448, 35.00000000000000000 ) ;
#15177=CIRCLE ( 'NONE', #5312, 5.000000000000000000 ) ;
#15179=ORIENTED_EDGE ( 'NONE', *, *, #6854, .F. ) ;
#15192=CARTESIAN_POINT ( 'NONE',  ( 1.352544480119999948, -20.86379603889999856, -146.5552959529999839 ) ) ;
#15209=CARTESIAN_POINT ( 'NONE',  ( -9.347107914279998653, -17.32706600430000066, -144.5552959529999839 ) ) ;
#15212=ORIENTED_EDGE ( 'NONE', *, *, #8806, .T. ) ;
#15218=ORIENTED_EDGE ( 'NONE', *, *, #13034, .T. ) ;
#15222=VECTOR ( 'NONE', #14592, 1000.000000000000000 ) ;
#15224=DIRECTION ( 'NONE',  ( -0.1435602414469281940, -0.9896415801065047146, 3.835814712303428266E-13 ) ) ;
#15225=CARTESIAN_POINT ( 'NONE',  ( 12.94820732169999999, -17.45719265660000019, -148.5552959529999839 ) ) ;
#15226=ORIENTED_EDGE ( 'NONE', *, *, #15047, .F. ) ;
#15231=DIRECTION ( 'NONE',  ( -0.9850838563818458127, 0.1720749717299729642, 4.465905845959301396E-12 ) ) ;
#15232=ORIENTED_EDGE ( 'NONE', *, *, #2358, .T. ) ;
#15236=EDGE_LOOP ( 'NONE', ( #12350, #8967, #16075, #18894, #9685, #8146 ) ) ;
#15237=FACE_OUTER_BOUND ( 'NONE', #17644, .T. ) ;
#15246=CARTESIAN_POINT ( 'NONE',  ( 23.41308733940000053, -15.43505800149999985, -148.5552959529999839 ) ) ;
#15249=PLANE ( 'NONE',  #8556 ) ;
#15258=CARTESIAN_POINT ( 'NONE',  ( 16.22102609572369758, -22.92413991441253529, -146.5552959530244834 ) ) ;
#15282=ORIENTED_EDGE ( 'NONE', *, *, #20813, .T. ) ;
#15313=EDGE_CURVE ( 'NONE', #2866, #10602, #1023, .T. ) ;
#15318=( GEOMETRIC_REPRESENTATION_CONTEXT ( 3 ) GLOBAL_UNCERTAINTY_ASSIGNED_CONTEXT ( ( #7081 ) ) GLOBAL_UNIT_ASSIGNED_CONTEXT ( ( #23244, #17651, #15858 ) ) REPRESENTATION_CONTEXT ( 'NONE', 'WORKASPACE' ) );
#15319=CARTESIAN_POINT ( 'NONE',  ( 17.33131581010000133, -22.98361965280000163, -147.5552959529999839 ) ) ;
#15337=VECTOR ( 'NONE', #14470, 1000.000000000000227 ) ;
#15344=CYLINDRICAL_SURFACE ( 'NONE', #2639, 9.999999999999998224 ) ;
#15346=CARTESIAN_POINT ( 'NONE',  ( 17.06104532839999877, -32.02344838739999489, -143.0552959529999839 ) ) ;
#15347=ORIENTED_EDGE ( 'NONE', *, *, #10821, .F. ) ;
#15353=CARTESIAN_POINT ( 'NONE',  ( 1.600095057559999923, -18.40127899619999852, -145.5552959529999839 ) ) ;
#15360=ORIENTED_EDGE ( 'NONE', *, *, #15793, .T. ) ;
#15362=DIRECTION ( 'NONE',  ( -0.1809478134909354996, 0.9834926989016490317, 9.461363557886634012E-13 ) ) ;
#15365=DIRECTION ( 'NONE',  ( 1.000000000000000000, 0.000000000000000000, -1.526556658859589738E-13 ) ) ;
#15372=CARTESIAN_POINT ( 'NONE',  ( -6.547730170579999509, -18.66441632429999942, -147.5552959529999839 ) ) ;
#15375=LINE ( 'NONE', #13111, #22149 ) ;
#15380=DIRECTION ( 'NONE',  ( 4.430318231639999944E-12, -6.100259101500000139E-13, 1.000000000000000000 ) ) ;
#15383=CARTESIAN_POINT ( 'NONE',  ( -9.334216945200001447, -17.19633444960000190, -146.5552959529999839 ) ) ;
#15395=CARTESIAN_POINT ( 'NONE',  ( 23.50000000000000000, -20.50000000000000000, -142.5552959529999839 ) ) ;
#15413=ORIENTED_EDGE ( 'NONE', *, *, #18244, .T. ) ;
#15415=ORIENTED_EDGE ( 'NONE', *, *, #9356, .T. ) ;
#15416=EDGE_CURVE ( 'NONE', #6279, #7923, #21010, .T. ) ;
#15422=ORIENTED_EDGE ( 'NONE', *, *, #17057, .F. ) ;
#15423=FACE_OUTER_BOUND ( 'NONE', #19144, .T. ) ;
#15430=VECTOR ( 'NONE', #8249, 1000.000000000000227 ) ;
#15433=DIRECTION ( 'NONE',  ( -0.1435602414469281940, -0.9896415801065048257, 3.847089866708073804E-13 ) ) ;
#15439=FACE_OUTER_BOUND ( 'NONE', #10677, .T. ) ;
#15442=DIRECTION ( 'NONE',  ( -0.9753087663813413410, 0.2208456705930775810, 8.936242978303132921E-12 ) ) ;
#15448=EDGE_LOOP ( 'NONE', ( #14507, #17897, #6500 ) ) ;
#15451=VERTEX_POINT ( 'NONE', #17070 ) ;
#15452=LINE ( 'NONE', #17602, #14796 ) ;
#15454=ORIENTED_EDGE ( 'NONE', *, *, #3080, .F. ) ;
#15458=CARTESIAN_POINT ( 'NONE',  ( 1.600095057559999923, -18.40127899619999852, -146.5552959529999839 ) ) ;
#15459=EDGE_CURVE ( 'NONE', #2337, #19493, #21369, .T. ) ;
#15466=DIRECTION ( 'NONE',  ( 0.9985681355238719137, -0.05349466063429310358, -4.511742413209420161E-12 ) ) ;
#15468=FACE_OUTER_BOUND ( 'NONE', #7568, .T. ) ;
#15471=FACE_OUTER_BOUND ( 'NONE', #13673, .T. ) ;
#15486=PLANE ( 'NONE',  #5049 ) ;
#15489=VERTEX_POINT ( 'NONE', #15874 ) ;
#15493=CARTESIAN_POINT ( 'NONE',  ( -9.347107914279998653, -17.32706600430000066, -143.5552959529999839 ) ) ;
#15502=LINE ( 'NONE', #20990, #3012 ) ;
#15505=EDGE_CURVE ( 'NONE', #17357, #21983, #23376, .T. ) ;
#15528=AXIS2_PLACEMENT_3D ( 'NONE', #11969, #15551, #6737 ) ;
#15536=VECTOR ( 'NONE', #14855, 1000.000000000000000 ) ;
#15549=ORIENTED_EDGE ( 'NONE', *, *, #737, .F. ) ;
#15551=DIRECTION ( 'NONE',  ( 8.955190032050000935E-12, -9.104778821549999739E-13, 1.000000000000000000 ) ) ;
#15553=ADVANCED_FACE ( 'NONE', ( #3266 ), #14215, .F. ) ;
#15563=VECTOR ( 'NONE', #93, 1000.000000000000114 ) ;
#15588=ORIENTED_EDGE ( 'NONE', *, *, #1037, .T. ) ;
#15591=CARTESIAN_POINT ( 'NONE',  ( 8.982728679470000088, -17.28848751049999777, -144.0552959529999839 ) ) ;
#15601=CARTESIAN_POINT ( 'NONE',  ( 5.792747474889999637, -16.92794981449999980, -144.5552959529999839 ) ) ;
#15606=DIRECTION ( 'NONE',  ( -0.9892101392001055871, 0.1465035852930155202, 0.000000000000000000 ) ) ;
#15608=DIRECTION ( 'NONE',  ( 0.9996028016287901163, -0.02818224575639410520, -1.295785648389728035E-13 ) ) ;
#15609=VECTOR ( 'NONE', #20065, 999.9999999999998863 ) ;
#15637=CARTESIAN_POINT ( 'NONE',  ( 16.16922456049999823, -22.27514461170000004, -148.5552959529999839 ) ) ;
#15638=EDGE_CURVE ( 'NONE', #11545, #760, #19462, .T. ) ;
#15655=DIRECTION ( 'NONE',  ( 1.526468026909924924E-13, 8.159623473500010254E-13, 1.000000000000000000 ) ) ;
#15664=VERTEX_POINT ( 'NONE', #5633 ) ;
#15676=CARTESIAN_POINT ( 'NONE',  ( -9.282104535849999394, -16.71402168319999859, -144.5552959529999839 ) ) ;
#15680=DIRECTION ( 'NONE',  ( 1.000000000000000000, 0.000000000000000000, -4.510774274160000731E-12 ) ) ;
#15686=ORIENTED_EDGE ( 'NONE', *, *, #17667, .F. ) ;
#15697=EDGE_CURVE ( 'NONE', #2813, #15749, #16240, .T. ) ;
#15700=DIRECTION ( 'NONE',  ( 4.430233957459999899E-12, -6.092903959140000514E-13, 1.000000000000000000 ) ) ;
#15708=CARTESIAN_POINT ( 'NONE',  ( 17.21087225569999646, -22.66053313549999970, -144.5552959529999839 ) ) ;
#15710=LINE ( 'NONE', #19159, #2290 ) ;
#15718=ORIENTED_EDGE ( 'NONE', *, *, #7493, .F. ) ;
#15720=ADVANCED_FACE ( 'NONE', ( #12532 ), #10742, .F. ) ;
#15723=FACE_OUTER_BOUND ( 'NONE', #8903, .T. ) ;
#15725=CARTESIAN_POINT ( 'NONE',  ( 5.631397321050000571, -17.85059010000000157, -146.5552959529999839 ) ) ;
#15737=CARTESIAN_POINT ( 'NONE',  ( 22.37638267690557115, -15.34326802965495773, -144.5552959530006945 ) ) ;
#15744=AXIS2_PLACEMENT_3D ( 'NONE', #16711, #7885, #14932 ) ;
#15746=SHAPE_REPRESENTATION ( 'Lock Tumblers', ( #5025 ), #13402 ) ;
#15749=VERTEX_POINT ( 'NONE', #287 ) ;
#15765=DIRECTION ( 'NONE',  ( 1.000000000000000000, 0.000000000000000000, -4.430318231639999944E-12 ) ) ;
#15767=CARTESIAN_POINT ( 'NONE',  ( 2.218297500549999857, -15.44723318490000175, -147.0552959529999839 ) ) ;
#15776=CARTESIAN_POINT ( 'NONE',  ( -5.758148842630000708, -13.22138763369999914, -147.5552959529999839 ) ) ;
#15778=ORIENTED_EDGE ( 'NONE', *, *, #6869, .T. ) ;
#15779=VERTEX_POINT ( 'NONE', #16357 ) ;
#15785=EDGE_CURVE ( 'NONE', #1140, #9187, #64, .T. ) ;
#15786=CARTESIAN_POINT ( 'NONE',  ( 1.807537990517430693, -16.33773399031227314, -145.5552959529913437 ) ) ;
#15789=VECTOR ( 'NONE', #22508, 1000.000000000000114 ) ;
#15790=FACE_OUTER_BOUND ( 'NONE', #8535, .T. ) ;
#15793=EDGE_CURVE ( 'NONE', #2929, #21873, #5980, .T. ) ;
#15800=ORIENTED_EDGE ( 'NONE', *, *, #14481, .T. ) ;
#15809=AXIS2_PLACEMENT_3D ( 'NONE', #1303, #1058, #6867 ) ;
#15810=CARTESIAN_POINT ( 'NONE',  ( -0.6781431574050000854, -62.17334590100000469, -148.0552959529999839 ) ) ;
#15816=ORIENTED_EDGE ( 'NONE', *, *, #9701, .F. ) ;
#15823=ORIENTED_EDGE ( 'NONE', *, *, #7065, .T. ) ;
#15832=CARTESIAN_POINT ( 'NONE',  ( -9.347107914279998653, -17.32706600430000066, -144.5552959529999839 ) ) ;
#15834=CARTESIAN_POINT ( 'NONE',  ( 23.93638409349999918, -31.59322175579999836, -144.0552959529999839 ) ) ;
#15837=DIRECTION ( 'NONE',  ( 4.510774274156380201E-12, -1.321907670943998010E-13, 1.000000000000000000 ) ) ;
#15842=DIRECTION ( 'NONE',  ( -0.1778629393740580045, -0.9840552701943220404, 3.562475540061165072E-13 ) ) ;
#15846=ADVANCED_FACE ( 'NONE', ( #2439 ), #2544, .F. ) ;
#15850=VERTEX_POINT ( 'NONE', #11448 ) ;
#15852=EDGE_CURVE ( 'NONE', #14794, #4187, #9767, .T. ) ;
#15858=( NAMED_UNIT ( * ) SI_UNIT ( $, .STERADIAN. ) SOLID_ANGLE_UNIT ( ) );
#15865=FACE_OUTER_BOUND ( 'NONE', #12646, .T. ) ;
#15869=DIRECTION ( 'NONE',  ( 0.7401352420267017784, 0.6724580459107286634, -3.250177904590145368E-12 ) ) ;
#15874=CARTESIAN_POINT ( 'NONE',  ( 16.52685120005601149, -19.88477712180281998, -143.5552959530023145 ) ) ;
#15875=LINE ( 'NONE', #23145, #8600 ) ;
#15883=VECTOR ( 'NONE', #22269, 1000.000000000000114 ) ;
#15888=DIRECTION ( 'NONE',  ( -8.956391184260000029E-12, 9.094947017729999296E-13, -1.000000000000000000 ) ) ;
#15889=CARTESIAN_POINT ( 'NONE',  ( -8.594304764349999459, -10.75357442870000035, -144.5552959529999839 ) ) ;
#15895=CARTESIAN_POINT ( 'NONE',  ( 24.75935218339999722, -28.32938697159999819, -146.5552959529999839 ) ) ;
#15901=CIRCLE ( 'NONE', #21994, 35.00000000000000000 ) ;
#15903=AXIS2_PLACEMENT_3D ( 'NONE', #14664, #5066, #4948 ) ;
#15909=ORIENTED_EDGE ( 'NONE', *, *, #11522, .F. ) ;
#15928=VECTOR ( 'NONE', #5824, 1000.000000000000000 ) ;
#15932=ORIENTED_EDGE ( 'NONE', *, *, #5745, .T. ) ;
#15937=ORIENTED_EDGE ( 'NONE', *, *, #5828, .T. ) ;
#15943=LINE ( 'NONE', #12355, #3031 ) ;
#15946=DIRECTION ( 'NONE',  ( -0.1000233216789610108, -0.9949850929136109245, 3.591470555298595137E-13 ) ) ;
#15948=LINE ( 'NONE', #12015, #21290 ) ;
#15956=FACE_OUTER_BOUND ( 'NONE', #6895, .T. ) ;
#15960=CARTESIAN_POINT ( 'NONE',  ( 4.468795199060000556, -26.40504320680000205, -142.5552959529999839 ) ) ;
#15971=CARTESIAN_POINT ( 'NONE',  ( -10.01911575600000148, -21.69748113039999637, -148.0552959529999839 ) ) ;
#15978=CARTESIAN_POINT ( 'NONE',  ( 23.99773978629999860, -29.25880395889999974, -147.5552959529999839 ) ) ;
#15980=ORIENTED_EDGE ( 'NONE', *, *, #12099, .T. ) ;
#15984=ORIENTED_EDGE ( 'NONE', *, *, #18567, .T. ) ;
#15988=VERTEX_POINT ( 'NONE', #2896 ) ;
#15994=PLANE ( 'NONE',  #20110 ) ;
#16001=CARTESIAN_POINT ( 'NONE',  ( -9.934356875269999776, -23.16624500709999879, -146.5552959529999839 ) ) ;
#16013=AXIS2_PLACEMENT_3D ( 'NONE', #2871, #20837, #8093 ) ;
#16014=VECTOR ( 'NONE', #7774, 1000.000000000000000 ) ;
#16022=EDGE_CURVE ( 'NONE', #12006, #20679, #10100, .T. ) ;
#16025=CARTESIAN_POINT ( 'NONE',  ( 22.40528270640000130, -21.39206583629999869, -146.5552959529999839 ) ) ;
#16032=VECTOR ( 'NONE', #11739, 1000.000000000000000 ) ;
#16033=ORIENTED_EDGE ( 'NONE', *, *, #8774, .F. ) ;
#16034=AXIS2_PLACEMENT_3D ( 'NONE', #14691, #20184, #11334 ) ;
#16035=DIRECTION ( 'NONE',  ( 1.000000000000000000, 0.000000000000000000, -1.527536832333224173E-13 ) ) ;
#16040=DIRECTION ( 'NONE',  ( -0.1000233216789610108, -0.9949850929136109245, 3.576398436658600095E-13 ) ) ;
#16047=PRODUCT_DEFINITION_SHAPE ( 'NONE', 'NONE',  #16194 ) ;
#16049=CARTESIAN_POINT ( 'NONE',  ( 16.26251912989999937, -22.62374141290000296, -144.5552959529999839 ) ) ;
#16060=LINE ( 'NONE', #5352, #272 ) ;
#16061=DIRECTION ( 'NONE',  ( -0.1000233216789610108, -0.9949850929136109245, 3.600083194518594546E-13 ) ) ;
#16068=AXIS2_PLACEMENT_3D ( 'NONE', #23159, #6732, #6853 ) ;
#16069=EDGE_CURVE ( 'NONE', #2852, #919, #19659, .T. ) ;
#16072=DIRECTION ( 'NONE',  ( 0.06298685227120542907, 0.9980143568310855251, -1.492139745100128694E-13 ) ) ;
#16075=ORIENTED_EDGE ( 'NONE', *, *, #13677, .T. ) ;
#16077=CARTESIAN_POINT ( 'NONE',  ( 16.74346552629999962, -18.31657829129999726, -148.5552959529999839 ) ) ;
#16081=FACE_OUTER_BOUND ( 'NONE', #22561, .T. ) ;
#16098=EDGE_CURVE ( 'NONE', #19591, #4852, #17335, .T. ) ;
#16105=( LENGTH_UNIT ( ) NAMED_UNIT ( * ) SI_UNIT ( .MILLI., .METRE. ) );
#16109=FACE_OUTER_BOUND ( 'NONE', #13090, .T. ) ;
#16110=PLANE ( 'NONE',  #10330 ) ;
#16118=DIRECTION ( 'NONE',  ( 1.000000000000000000, 0.000000000000000000, -2.715621035259064790E-14 ) ) ;
#16121=VECTOR ( 'NONE', #15608, 1000.000000000000114 ) ;
#16128=EDGE_LOOP ( 'NONE', ( #2193, #4689, #6408, #11623, #8310, #15980, #4813, #16566, #14388, #15422 ) ) ;
#16149=DIRECTION ( 'NONE',  ( 1.000000000000000000, 0.000000000000000000, -2.854859206178974232E-14 ) ) ;
#16150=ORIENTED_EDGE ( 'NONE', *, *, #19842, .F. ) ;
#16153=CARTESIAN_POINT ( 'NONE',  ( 1.172620240290000115, -63.19354141059999108, -146.0552959529999839 ) ) ;
#16164=ORIENTED_EDGE ( 'NONE', *, *, #22861, .F. ) ;
#16172=DIRECTION ( 'NONE',  ( 1.000000000000000000, 0.000000000000000000, -1.498801083243961330E-13 ) ) ;
#16186=DIRECTION ( 'NONE',  ( 4.430318231639999944E-12, -6.100259101500000139E-13, 1.000000000000000000 ) ) ;
#16191=VECTOR ( 'NONE', #12770, 1000.000000000000114 ) ;
#16194=PRODUCT_DEFINITION ( 'UNKNOWN', '', #516, #5420 ) ;
#16201=DIRECTION ( 'NONE',  ( -0.06298685227120542907, -0.9980143568310855251, 1.515824502950130739E-13 ) ) ;
#16205=CIRCLE ( 'NONE', #6324, 8.176568160360000448 ) ;
#16214=EDGE_CURVE ( 'NONE', #2750, #15988, #10850, .T. ) ;
#16224=CARTESIAN_POINT ( 'NONE',  ( 5.792747474879999636, -16.92794981449999980, -145.5552959529999839 ) ) ;
#16228=EDGE_LOOP ( 'NONE', ( #17050, #3311, #8406 ) ) ;
#16233=EDGE_CURVE ( 'NONE', #21733, #16939, #13093, .T. ) ;
#16234=FACE_OUTER_BOUND ( 'NONE', #7565, .T. ) ;
#16237=DIRECTION ( 'NONE',  ( 2.842170943040000002E-14, 3.570477247189999985E-13, 1.000000000000000000 ) ) ;
#16240=LINE ( 'NONE', #3510, #18847 ) ;
#16252=CARTESIAN_POINT ( 'NONE',  ( 21.39890631740000160, -21.26106171180000359, -145.0552959529999839 ) ) ;
#16255=VECTOR ( 'NONE', #3479, 999.9999999999998863 ) ;
#16260=PLANE ( 'NONE',  #16068 ) ;
#16266=EDGE_CURVE ( 'NONE', #21497, #20668, #20481, .T. ) ;
#16278=ORIENTED_EDGE ( 'NONE', *, *, #7368, .T. ) ;
#16284=CARTESIAN_POINT ( 'NONE',  ( 16.26858689138171243, -22.56086829267852778, -144.5552959530247108 ) ) ;
#16287=LINE ( 'NONE', #8649, #9106 ) ;
#16288=DIRECTION ( 'NONE',  ( 0.1435602414469281940, 0.9896415801065048257, -3.836930773098079160E-13 ) ) ;
#16292=ORIENTED_EDGE ( 'NONE', *, *, #1766, .F. ) ;
#16296=VECTOR ( 'NONE', #14265, 1000.000000000000114 ) ;
#16297=ORIENTED_EDGE ( 'NONE', *, *, #22197, .T. ) ;
#16302=ORIENTED_EDGE ( 'NONE', *, *, #17107, .F. ) ;
#16305=PLANE ( 'NONE',  #14081 ) ;
#16306=CARTESIAN_POINT ( 'NONE',  ( -6.657076963140000636, -20.13603737529999904, -144.5552959529999839 ) ) ;
#16308=CARTESIAN_POINT ( 'NONE',  ( 15.97954986339999905, -26.72957102550000030, -142.5552959529999839 ) ) ;
#16319=CARTESIAN_POINT ( 'NONE',  ( 8.995627988029999855, -17.23072307649999857, -146.0552959529999839 ) ) ;
#16341=DIRECTION ( 'NONE',  ( 0.000000000000000000, -1.000000000000000000, 3.568879590630000244E-13 ) ) ;
#16345=CIRCLE ( 'NONE', #6077, 5.000000000000000000 ) ;
#16346=ORIENTED_EDGE ( 'NONE', *, *, #23218, .F. ) ;
#16349=VECTOR ( 'NONE', #6647, 1000.000000000000000 ) ;
#16352=VERTEX_POINT ( 'NONE', #19040 ) ;
#16354=DIRECTION ( 'NONE',  ( 1.000000000000000000, 0.000000000000000000, -8.955190032050000935E-12 ) ) ;
#16357=CARTESIAN_POINT ( 'NONE',  ( 23.08797222880000177, -15.45109671570000032, -142.5552959529999839 ) ) ;
#16367=EDGE_CURVE ( 'NONE', #19736, #4115, #6542, .T. ) ;
#16372=CARTESIAN_POINT ( 'NONE',  ( -4.888913597060000171, -24.24628707910000003, -143.5552959529999839 ) ) ;
#16377=ADVANCED_FACE ( 'NONE', ( #3102 ), #8658, .T. ) ;
#16379=DIRECTION ( 'NONE',  ( 1.526468026909999897E-13, 8.159623473500000156E-13, 1.000000000000000000 ) ) ;
#16382=DIRECTION ( 'NONE',  ( 0.000000000000000000, 3.900299903225544950E-11, -1.000000000000000000 ) ) ;
#16386=LINE ( 'NONE', #3297, #15563 ) ;
#16389=ORIENTED_EDGE ( 'NONE', *, *, #21188, .T. ) ;
#16404=DIRECTION ( 'NONE',  ( -0.9753087663813413410, 0.2208456705930775810, 8.935806277123132252E-12 ) ) ;
#16405=LINE ( 'NONE', #3558, #3895 ) ;
#16407=CARTESIAN_POINT ( 'NONE',  ( -9.282104535860000283, -16.71402168319999859, -145.5552959529999839 ) ) ;
#16413=CIRCLE ( 'NONE', #11462, 8.176568160360000448 ) ;
#16419=CARTESIAN_POINT ( 'NONE',  ( -5.070907855439999778, -22.41528233759999722, -148.0552959529999839 ) ) ;
#16425=CARTESIAN_POINT ( 'NONE',  ( -6.601136089949999786, -20.10368962670000315, -143.5552959529999839 ) ) ;
#16429=CIRCLE ( 'NONE', #7302, 35.00000000000000000 ) ;
#16431=CIRCLE ( 'NONE', #118, 8.176568160360000448 ) ;
#16436=DIRECTION ( 'NONE',  ( -0.1146332952500066227, -0.9934078757590583120, -9.710750722050572275E-14 ) ) ;
#16438=ORIENTED_EDGE ( 'NONE', *, *, #2842, .F. ) ;
#16439=CARTESIAN_POINT ( 'NONE',  ( -2.718705559363074897, -28.41053430194196494, -145.5552959530122905 ) ) ;
#16452=ADVANCED_FACE ( 'NONE', ( #1324 ), #23085, .T. ) ;
#16456=DIRECTION ( 'NONE',  ( -0.1000233216789610108, -0.9949850929136109245, 3.591470555298595137E-13 ) ) ;
#16460=ORIENTED_EDGE ( 'NONE', *, *, #14141, .T. ) ;
#16462=VERTEX_POINT ( 'NONE', #12242 ) ;
#16474=EDGE_LOOP ( 'NONE', ( #7773, #21747, #19243, #20499 ) ) ;
#16490=EDGE_CURVE ( 'NONE', #16855, #9023, #7130, .T. ) ;
#16500=ORIENTED_EDGE ( 'NONE', *, *, #3145, .F. ) ;
#16503=ORIENTED_EDGE ( 'NONE', *, *, #17660, .T. ) ;
#16516=DIRECTION ( 'NONE',  ( -0.1465035852930155202, -0.9892101392001055871, 4.561368942930487546E-14 ) ) ;
#16518=ORIENTED_EDGE ( 'NONE', *, *, #3159, .F. ) ;
#16522=EDGE_CURVE ( 'NONE', #1779, #2894, #19983, .T. ) ;
#16537=ORIENTED_EDGE ( 'NONE', *, *, #744, .T. ) ;
#16544=EDGE_LOOP ( 'NONE', ( #4804, #13813, #8971 ) ) ;
#16548=EDGE_CURVE ( 'NONE', #5742, #473, #21786, .T. ) ;
#16555=ORIENTED_EDGE ( 'NONE', *, *, #19127, .T. ) ;
#16559=FACE_OUTER_BOUND ( 'NONE', #20313, .T. ) ;
#16562=CARTESIAN_POINT ( 'NONE',  ( 16.65421564080000039, -18.61497348660000029, -146.5552959529999839 ) ) ;
#16565=PLANE ( 'NONE',  #21444 ) ;
#16566=ORIENTED_EDGE ( 'NONE', *, *, #10708, .F. ) ;
#16570=ORIENTED_EDGE ( 'NONE', *, *, #21864, .F. ) ;
#16572=EDGE_CURVE ( 'NONE', #23456, #2031, #14628, .T. ) ;
#16574=CARTESIAN_POINT ( 'NONE',  ( 25.15155135439999867, -26.08415009650000016, -147.0552959529999839 ) ) ;
#16597=VECTOR ( 'NONE', #19660, 999.9999999999998863 ) ;
#16604=ORIENTED_EDGE ( 'NONE', *, *, #16732, .T. ) ;
#16616=ORIENTED_EDGE ( 'NONE', *, *, #12285, .F. ) ;
#16619=ORIENTED_EDGE ( 'NONE', *, *, #14694, .T. ) ;
#16620=CARTESIAN_POINT ( 'NONE',  ( 24.35183050010000017, -28.38413933620000051, -145.5552959529999839 ) ) ;
#16622=CARTESIAN_POINT ( 'NONE',  ( -9.334216945200001447, -17.19633444960000190, -145.5552959529999839 ) ) ;
#16625=ORIENTED_EDGE ( 'NONE', *, *, #7751, .F. ) ;
#16630=DIRECTION ( 'NONE',  ( 1.526468026909999897E-13, 8.159623473500000156E-13, 1.000000000000000000 ) ) ;
#16642=ORIENTED_EDGE ( 'NONE', *, *, #12600, .F. ) ;
#16647=ORIENTED_EDGE ( 'NONE', *, *, #3565, .F. ) ;
#16650=ADVANCED_FACE ( 'NONE', ( #3271 ), #21132, .T. ) ;
#16657=EDGE_CURVE ( 'NONE', #10871, #6792, #14103, .T. ) ;
#16683=CARTESIAN_POINT ( 'NONE',  ( -6.370493725010000219, -17.65251768590000125, -144.5552959529999839 ) ) ;
#16684=AXIS2_PLACEMENT_3D ( 'NONE', #15493, #9887, #20858 ) ;
#16685=ORIENTED_EDGE ( 'NONE', *, *, #6911, .F. ) ;
#16704=ORIENTED_EDGE ( 'NONE', *, *, #20447, .F. ) ;
#16705=ADVANCED_FACE ( 'NONE', ( #21487 ), #19689, .F. ) ;
#16706=VECTOR ( 'NONE', #19637, 1000.000000000000114 ) ;
#16711=CARTESIAN_POINT ( 'NONE',  ( 22.40884248670000289, -21.39641658300000060, -143.5552959529999839 ) ) ;
#16713=DIRECTION ( 'NONE',  ( 1.527666881879999979E-13, 8.153477892850000134E-13, 1.000000000000000000 ) ) ;
#16715=CARTESIAN_POINT ( 'NONE',  ( -9.334216945200001447, -17.19633444960000190, -145.5552959529999839 ) ) ;
#16716=VERTEX_POINT ( 'NONE', #5287 ) ;
#16720=VECTOR ( 'NONE', #17063, 999.9999999999998863 ) ;
#16729=ORIENTED_EDGE ( 'NONE', *, *, #13766, .T. ) ;
#16732=EDGE_CURVE ( 'NONE', #7451, #7250, #19466, .T. ) ;
#16739=VECTOR ( 'NONE', #14878, 1000.000000000000227 ) ;
#16766=FACE_OUTER_BOUND ( 'NONE', #5875, .T. ) ;
#16768=ORIENTED_EDGE ( 'NONE', *, *, #7751, .T. ) ;
#16777=CLOSED_SHELL ( 'NONE', ( #15720, #12563, #10241, #21755, #5662, #20409, #14933, #2781, #1385, #9503, #20913, #17817, #8480, #20071, #6608, #22739, #18454, #11410, #3508, #12887, #9600, #2998, #19023, #16452, #4818, #22774, #4310, #13570, #6559, #22533, #13321, #22026, #5279, #13005, #4628, #5207, #11455, #799, #9676, #17194, #7057, #17939, #9199, #10813, #8462, #23273, #21153, #7845, #4171, #13084, #21935, #1992, #21741, #5464, #15553, #6711, #512, #9093, #14488, #7899, #1851, #475, #1817, #10890, #13582, #5667, #14349, #11253, #14403, #16377, #12781, #12410, #4219, #19154, #9669, #11826, #2354, #3611, #12561, #3267, #4002, #821, #20857, #8191, #21749, #19690, #5322, #440, #9409, #22494, #5539, #10893, #332, #2823, #13887, #2091, #17247, #5468, #16650, #8080, #19065, #1739, #22185, #15846, #12482, #16705, #6038, #5879, #17967, #17252, #2973, #22846, #6794, #12687, #21611, #12584, #6528, #22273, #3738, #20888, #17522, #13769, #222, #19515, #8685, #14782, #17810, #4572, #20376, #16867, #14895, #13759, #2806, #11639, #7968, #4308, #19517, #13178, #9655, #5323, #13080, #7199, #14159 ) ) ;
#16792=VERTEX_POINT ( 'NONE', #19929 ) ;
#16793=VECTOR ( 'NONE', #18329, 1000.000000000000114 ) ;
#16795=CARTESIAN_POINT ( 'NONE',  ( -7.149448239889999890, -25.45628515800000002, -145.5552959529999839 ) ) ;
#16803=PLANE ( 'NONE',  #18317 ) ;
#16804=DIRECTION ( 'NONE',  ( 1.000000000000000000, 0.000000000000000000, -1.498801083243961330E-13 ) ) ;
#16812=AXIS2_PLACEMENT_3D ( 'NONE', #15810, #20817, #11877 ) ;
#16814=DIRECTION ( 'NONE',  ( 4.510774274160000731E-12, -1.321907670990000086E-13, 1.000000000000000000 ) ) ;
#16818=DIRECTION ( 'NONE',  ( 0.000000000000000000, -1.000000000000000000, 3.568879590630000244E-13 ) ) ;
#16834=CARTESIAN_POINT ( 'NONE',  ( -9.934356875269999776, -23.16624500709999879, -146.0552959529999839 ) ) ;
#16836=EDGE_LOOP ( 'NONE', ( #4589, #7295, #2681, #11812, #9712, #10588, #21513 ) ) ;
#16838=LINE ( 'NONE', #6120, #16720 ) ;
#16847=VERTEX_POINT ( 'NONE', #11325 ) ;
#16855=VERTEX_POINT ( 'NONE', #10984 ) ;
#16858=ORIENTED_EDGE ( 'NONE', *, *, #3963, .F. ) ;
#16867=ADVANCED_FACE ( 'NONE', ( #5416 ), #12774, .T. ) ;
#16868=EDGE_CURVE ( 'NONE', #22098, #12475, #1977, .T. ) ;
#16870=CARTESIAN_POINT ( 'NONE',  ( 2.048233066679999936, -63.64014441970000746, -143.5552959529999839 ) ) ;
#16876=FACE_OUTER_BOUND ( 'NONE', #4740, .T. ) ;
#16879=DIRECTION ( 'NONE',  ( 0.1824094679249879947, 0.9832226533249336375, -8.292396948119437334E-13 ) ) ;
#16882=LINE ( 'NONE', #16425, #20605 ) ;
#16886=ORIENTED_EDGE ( 'NONE', *, *, #1766, .T. ) ;
#16905=CARTESIAN_POINT ( 'NONE',  ( 22.01137100460000084, -15.39610142400000115, -146.5552959529999839 ) ) ;
#16920=CARTESIAN_POINT ( 'NONE',  ( 15.87827223000000032, -26.60524292859999917, -143.5552959529999839 ) ) ;
#16924=VECTOR ( 'NONE', #13364, 1000.000000000000000 ) ;
#16928=VERTEX_POINT ( 'NONE', #20747 ) ;
#16937=CARTESIAN_POINT ( 'NONE',  ( 12.01554901919999985, -37.47280209340000567, -145.5552959529999839 ) ) ;
#16939=VERTEX_POINT ( 'NONE', #20992 ) ;
#16942=CARTESIAN_POINT ( 'NONE',  ( -9.347107914279998653, -17.32706600430000066, -144.5552959529999839 ) ) ;
#16947=LINE ( 'NONE', #7547, #13682 ) ;
#16949=EDGE_CURVE ( 'NONE', #11927, #15664, #11801, .T. ) ;
#16957=AXIS2_PLACEMENT_3D ( 'NONE', #9514, #7617, #18349 ) ;
#16962=CARTESIAN_POINT ( 'NONE',  ( -6.384923429577490595, -17.86333053711281238, -143.5552959530020303 ) ) ;
#16972=DIRECTION ( 'NONE',  ( -0.1435602414469281940, -0.9896415801065048257, 3.836930773098079160E-13 ) ) ;
#16973=EDGE_CURVE ( 'NONE', #8373, #9593, #20514, .T. ) ;
#16986=LINE ( 'NONE', #6163, #2950 ) ;
#16994=FACE_OUTER_BOUND ( 'NONE', #9496, .T. ) ;
#16998=ORIENTED_EDGE ( 'NONE', *, *, #792, .T. ) ;
#17006=AXIS2_PLACEMENT_3D ( 'NONE', #8470, #23233, #19787 ) ;
#17011=ORIENTED_EDGE ( 'NONE', *, *, #10335, .T. ) ;
#17016=DIRECTION ( 'NONE',  ( -0.1743118874569385135, -0.9846904924346531196, 6.644571628977660906E-13 ) ) ;
#17019=CARTESIAN_POINT ( 'NONE',  ( 1.759100530420000030, -16.38142836440000139, -143.0552959529999839 ) ) ;
#17021=FACE_OUTER_BOUND ( 'NONE', #17824, .T. ) ;
#17026=EDGE_CURVE ( 'NONE', #4889, #18609, #890, .T. ) ;
#17028=CARTESIAN_POINT ( 'NONE',  ( 5.276897646260000130, -21.39828525539999760, -144.5552959529999839 ) ) ;
#17031=CARTESIAN_POINT ( 'NONE',  ( -6.049191701419999845, -14.51144913589999952, -145.5552959529999839 ) ) ;
#17037=AXIS2_PLACEMENT_3D ( 'NONE', #20851, #6325, #7329 ) ;
#17040=PLANE ( 'NONE',  #16684 ) ;
#17050=ORIENTED_EDGE ( 'NONE', *, *, #22849, .F. ) ;
#17054=ORIENTED_EDGE ( 'NONE', *, *, #8631, .T. ) ;
#17057=EDGE_CURVE ( 'NONE', #6997, #7250, #18732, .T. ) ;
#17059=VECTOR ( 'NONE', #23505, 999.9999999999998863 ) ;
#17063=DIRECTION ( 'NONE',  ( -0.09606172499277226828, -0.9953753789357124848, 8.265980492677616040E-13 ) ) ;
#17069=VECTOR ( 'NONE', #12092, 1000.000000000000227 ) ;
#17070=CARTESIAN_POINT ( 'NONE',  ( -9.056357402059999728, -12.43025388040000045, -146.5552959529999839 ) ) ;
#17073=ORIENTED_EDGE ( 'NONE', *, *, #513, .T. ) ;
#17074=VECTOR ( 'NONE', #10298, 1000.000000000000114 ) ;
#17081=FACE_OUTER_BOUND ( 'NONE', #12897, .T. ) ;
#17084=DIRECTION ( 'NONE',  ( 0.000000000000000000, 0.000000000000000000, 1.000000000000000000 ) ) ;
#17086=CARTESIAN_POINT ( 'NONE',  ( -6.370493725020000220, -17.65251768590000125, -145.5552959529999839 ) ) ;
#17091=EDGE_LOOP ( 'NONE', ( #10750, #3649 ) ) ;
#17093=CARTESIAN_POINT ( 'NONE',  ( -9.394779979509999990, -17.86685386420000299, -143.5552959529999839 ) ) ;
#17096=VECTOR ( 'NONE', #16713, 1000.000000000000000 ) ;
#17098=AXIS2_PLACEMENT_3D ( 'NONE', #15776, #6610, #2584 ) ;
#17101=ORIENTED_EDGE ( 'NONE', *, *, #98, .T. ) ;
#17104=CARTESIAN_POINT ( 'NONE',  ( -6.599319970649999867, -19.98386714700000155, -145.5552959529999839 ) ) ;
#17105=EDGE_LOOP ( 'NONE', ( #8055, #4576, #2208, #9110, #17011, #3827, #9881, #14310, #8609, #13546 ) ) ;
#17107=EDGE_CURVE ( 'NONE', #15489, #21292, #12041, .T. ) ;
#17110=EDGE_LOOP ( 'NONE', ( #6097, #16297, #20252, #23529, #15454, #22698, #16164 ) ) ;
#17112=CARTESIAN_POINT ( 'NONE',  ( 16.64676602990000021, -18.64223989710000140, -143.5552959529999839 ) ) ;
#17116=FACE_OUTER_BOUND ( 'NONE', #20418, .T. ) ;
#17121=ORIENTED_EDGE ( 'NONE', *, *, #20371, .F. ) ;
#17125=PLANE ( 'NONE',  #21254 ) ;
#17126=FACE_OUTER_BOUND ( 'NONE', #20411, .T. ) ;
#17127=ORIENTED_EDGE ( 'NONE', *, *, #7490, .F. ) ;
#17130=CARTESIAN_POINT ( 'NONE',  ( 1.342750202250000191, -63.28208324180000233, -144.5552959529999839 ) ) ;
#17136=EDGE_CURVE ( 'NONE', #2114, #3418, #8580, .T. ) ;
#17140=PLANE ( 'NONE',  #1900 ) ;
#17144=DIRECTION ( 'NONE',  ( 0.9968185442904002880, -0.07970438983373201447, -8.712538262633510059E-14 ) ) ;
#17151=CARTESIAN_POINT ( 'NONE',  ( 1.847645635000000119, -15.93876195360000025, -145.5552959529999839 ) ) ;
#17154=ORIENTED_EDGE ( 'NONE', *, *, #15047, .T. ) ;
#17156=DIRECTION ( 'NONE',  ( 1.000000000000000000, 0.000000000000000000, -1.522591576628786004E-13 ) ) ;
#17163=DIRECTION ( 'NONE',  ( 4.510170015240000199E-12, -1.314504061159999897E-13, 1.000000000000000000 ) ) ;
#17175=ORIENTED_EDGE ( 'NONE', *, *, #10824, .F. ) ;
#17194=ADVANCED_FACE ( 'NONE', ( #12163 ), #21458, .T. ) ;
#17195=AXIS2_PLACEMENT_3D ( 'NONE', #20383, #16379, #8102 ) ;
#17197=LINE ( 'NONE', #9802, #7524 ) ;
#17206=ORIENTED_EDGE ( 'NONE', *, *, #19294, .F. ) ;
#17213=EDGE_CURVE ( 'NONE', #9023, #5742, #22043, .T. ) ;
#17230=VERTEX_POINT ( 'NONE', #2523 ) ;
#17238=EDGE_CURVE ( 'NONE', #5977, #20549, #6086, .T. ) ;
#17243=DIRECTION ( 'NONE',  ( -1.296824736026760017E-11, 0.000000000000000000, 1.000000000000000000 ) ) ;
#17244=ORIENTED_EDGE ( 'NONE', *, *, #2419, .F. ) ;
#17246=ORIENTED_EDGE ( 'NONE', *, *, #7210, .T. ) ;
#17247=ADVANCED_FACE ( 'NONE', ( #15471 ), #7973, .F. ) ;
#17252=ADVANCED_FACE ( 'NONE', ( #11649 ), #15249, .T. ) ;
#17253=VECTOR ( 'NONE', #4928, 1000.000000000000000 ) ;
#17258=CARTESIAN_POINT ( 'NONE',  ( 1.708387416626109934, -17.47608414525880960, -147.5552959529822488 ) ) ;
#17260=ORIENTED_EDGE ( 'NONE', *, *, #6586, .F. ) ;
#17261=CARTESIAN_POINT ( 'NONE',  ( 8.633772787779999902, -29.00605602609999778, -146.5552959529999839 ) ) ;
#17266=LINE ( 'NONE', #6783, #11704 ) ;
#17267=ORIENTED_EDGE ( 'NONE', *, *, #2222, .T. ) ;
#17269=VECTOR ( 'NONE', #10354, 999.9999999999998863 ) ;
#17272=LINE ( 'NONE', #10236, #3894 ) ;
#17275=CARTESIAN_POINT ( 'NONE',  ( -9.874497313270580889, -24.62570111238803960, -143.5552959529987334 ) ) ;
#17286=DIRECTION ( 'NONE',  ( 2.839308199618490134E-14, 3.568879590628495223E-13, 1.000000000000000000 ) ) ;
#17292=EDGE_LOOP ( 'NONE', ( #13667, #8485, #5297, #9353 ) ) ;
#17298=EDGE_LOOP ( 'NONE', ( #15282, #10116, #20784, #13728, #451, #20210 ) ) ;
#17299=EDGE_CURVE ( 'NONE', #2628, #2618, #18926, .T. ) ;
#17300=CARTESIAN_POINT ( 'NONE',  ( 23.40529971389999986, -31.60139774330000151, -147.5552959529999839 ) ) ;
#17303=EDGE_CURVE ( 'NONE', #23020, #7470, #15006, .T. ) ;
#17305=LINE ( 'NONE', #1019, #9510 ) ;
#17319=CARTESIAN_POINT ( 'NONE',  ( 19.86977406280000125, -31.59375768830000197, -148.5552959529999839 ) ) ;
#17335=CIRCLE ( 'NONE', #18473, 9.999999999999998224 ) ;
#17339=DIRECTION ( 'NONE',  ( 4.430318231639999944E-12, -6.100259101500000139E-13, 1.000000000000000000 ) ) ;
#17346=CARTESIAN_POINT ( 'NONE',  ( 1.591914056710000080, -18.48847405160000079, -144.5552959529999839 ) ) ;
#17350=VECTOR ( 'NONE', #14736, 1000.000000000000114 ) ;
#17353=FACE_OUTER_BOUND ( 'NONE', #2739, .T. ) ;
#17357=VERTEX_POINT ( 'NONE', #18811 ) ;
#17368=CARTESIAN_POINT ( 'NONE',  ( -5.070907855429999778, -22.41528233759999722, -147.5552959529999839 ) ) ;
#17378=PLANE ( 'NONE',  #16013 ) ;
#17385=DIRECTION ( 'NONE',  ( 0.000000000000000000, -1.000000000000000000, 8.159623473500000156E-13 ) ) ;
#17390=ORIENTED_EDGE ( 'NONE', *, *, #18941, .F. ) ;
#17392=CARTESIAN_POINT ( 'NONE',  ( -9.434278515689999978, -18.41834002140000237, -146.5552959529999839 ) ) ;
#17411=SURFACE_SIDE_STYLE ('',( #19446 ) ) ;
#17414=CARTESIAN_POINT ( 'NONE',  ( 17.33131581010000133, -22.98361965280000163, -146.5552959529999839 ) ) ;
#17416=ORIENTED_EDGE ( 'NONE', *, *, #22147, .T. ) ;
#17417=CARTESIAN_POINT ( 'NONE',  ( 24.38136133040000075, -29.22855050349999928, -146.5552959529999839 ) ) ;
#17418=DIRECTION ( 'NONE',  ( 4.510774274160000731E-12, -1.321907670990000086E-13, 1.000000000000000000 ) ) ;
#17420=ORIENTED_EDGE ( 'NONE', *, *, #23077, .F. ) ;
#17423=DIRECTION ( 'NONE',  ( 0.9957290851625899553, -0.09232328504376198508, -9.001390970786290700E-12 ) ) ;
#17434=AXIS2_PLACEMENT_3D ( 'NONE', #21204, #6556, #17503 ) ;
#17435=ORIENTED_EDGE ( 'NONE', *, *, #22861, .T. ) ;
#17437=ORIENTED_EDGE ( 'NONE', *, *, #22602, .T. ) ;
#17438=AXIS2_PLACEMENT_3D ( 'NONE', #17130, #9506, #22373 ) ;
#17439=LINE ( 'NONE', #17086, #9444 ) ;
#17448=AXIS2_PLACEMENT_3D ( 'NONE', #16870, #22230, #580 ) ;
#17453=AXIS2_PLACEMENT_3D ( 'NONE', #12674, #14119, #17924 ) ;
#17472=EDGE_LOOP ( 'NONE', ( #11132, #17246, #1979, #3404, #22459, #11179, #11270, #1460, #1549, #20362 ) ) ;
#17476=ORIENTED_EDGE ( 'NONE', *, *, #1462, .F. ) ;
#17480=FACE_OUTER_BOUND ( 'NONE', #13021, .T. ) ;
#17488=COLOUR_RGB ( '', 0.66274510, 0.83137255, 0.94901961) ;
#17503=DIRECTION ( 'NONE',  ( 1.000000000000000000, 0.000000000000000000, -4.510774274160000731E-12 ) ) ;
#17520=EDGE_CURVE ( 'NONE', #1590, #9187, #19635, .T. ) ;
#17522=ADVANCED_FACE ( 'NONE', ( #14165 ), #8788, .F. ) ;
#17523=CARTESIAN_POINT ( 'NONE',  ( -6.601136089949999786, -20.10368962670000315, -144.5552959529999839 ) ) ;
#17531=LINE ( 'NONE', #1251, #9542 ) ;
#17543=DIRECTION ( 'NONE',  ( -0.9846904924346530086, 0.1743118874569384857, 8.976860394976840322E-12 ) ) ;
#17546=ORIENTED_EDGE ( 'NONE', *, *, #17303, .F. ) ;
#17547=VECTOR ( 'NONE', #6726, 1000.000000000000227 ) ;
#17566=AXIS2_PLACEMENT_3D ( 'NONE', #4895, #19416, #13698 ) ;
#17573=ORIENTED_EDGE ( 'NONE', *, *, #8919, .F. ) ;
#17578=EDGE_CURVE ( 'NONE', #10772, #1657, #1920, .T. ) ;
#17581=CARTESIAN_POINT ( 'NONE',  ( -9.157754307290000284, -15.75963164970000108, -147.5552959529999839 ) ) ;
#17587=ORIENTED_EDGE ( 'NONE', *, *, #10335, .F. ) ;
#17590=LINE ( 'NONE', #8524, #6765 ) ;
#17597=CARTESIAN_POINT ( 'NONE',  ( -4.160432423080000497, -28.71743394529999804, -144.0552959529999839 ) ) ;
#17602=CARTESIAN_POINT ( 'NONE',  ( -9.394779979509999990, -17.86685386420000299, -142.5552959529999839 ) ) ;
#17605=CARTESIAN_POINT ( 'NONE',  ( 1.561837858109999866, -18.84848306830000197, -142.5552959529999839 ) ) ;
#17608=LINE ( 'NONE', #6537, #3379 ) ;
#17612=DIRECTION ( 'NONE',  ( -0.9874789572432817186, 0.1577507813030449846, 2.125043109900604696E-14 ) ) ;
#17613=DIRECTION ( 'NONE',  ( -0.9934078757590584230, 0.1146332952500066366, 4.471042303700267278E-12 ) ) ;
#17632=CYLINDRICAL_SURFACE ( 'NONE', #3913, 6.000000000000002665 ) ;
#17635=EDGE_LOOP ( 'NONE', ( #16460, #1895, #13610, #18696, #124 ) ) ;
#17644=EDGE_LOOP ( 'NONE', ( #15415, #496, #11029, #20885, #101, #10830, #3748 ) ) ;
#17648=CARTESIAN_POINT ( 'NONE',  ( -9.282104535849999394, -16.71402168319999859, -144.5552959529999839 ) ) ;
#17651=( NAMED_UNIT ( * ) PLANE_ANGLE_UNIT ( ) SI_UNIT ( $, .RADIAN. ) );
#17660=EDGE_CURVE ( 'NONE', #7470, #5559, #9, .T. ) ;
#17663=CARTESIAN_POINT ( 'NONE',  ( 12.91075631260000023, -38.04527125359999928, -147.0552959529999839 ) ) ;
#17666=DIRECTION ( 'NONE',  ( 4.510774274160000731E-12, -1.321907670990000086E-13, 1.000000000000000000 ) ) ;
#17667=EDGE_CURVE ( 'NONE', #17230, #19591, #19988, .T. ) ;
#17671=VERTEX_POINT ( 'NONE', #10923 ) ;
#17676=ORIENTED_EDGE ( 'NONE', *, *, #3682, .F. ) ;
#17678=CARTESIAN_POINT ( 'NONE',  ( 7.085709294149999060, -13.66851965709999916, -142.5552959529999839 ) ) ;
#17682=VERTEX_POINT ( 'NONE', #9606 ) ;
#17683=DIRECTION ( 'NONE',  ( 1.526468026909999897E-13, 8.159623473500000156E-13, 1.000000000000000000 ) ) ;
#17686=FACE_OUTER_BOUND ( 'NONE', #19851, .T. ) ;
#17687=CARTESIAN_POINT ( 'NONE',  ( 23.40529971389999986, -31.60139774330000151, -148.5552959529999839 ) ) ;
#17694=VECTOR ( 'NONE', #4189, 1000.000000000000000 ) ;
#17696=VECTOR ( 'NONE', #18977, 1000.000000000000000 ) ;
#17699=VERTEX_POINT ( 'NONE', #20457 ) ;
#17712=CARTESIAN_POINT ( 'NONE',  ( 16.26251912989999937, -22.62374141290000296, -143.5552959529999839 ) ) ;
#17714=DIRECTION ( 'NONE',  ( 0.09606172499277226828, 0.9953753789357124848, -8.277822871607614780E-13 ) ) ;
#17715=ORIENTED_EDGE ( 'NONE', *, *, #17026, .T. ) ;
#17725=LINE ( 'NONE', #19404, #20894 ) ;
#17743=DIRECTION ( 'NONE',  ( 0.000000000000000000, -1.000000000000000000, 3.568879590630000244E-13 ) ) ;
#17746=ORIENTED_EDGE ( 'NONE', *, *, #7340, .T. ) ;
#17755=VECTOR ( 'NONE', #10186, 999.9999999999998863 ) ;
#17756=LINE ( 'NONE', #15978, #3733 ) ;
#17762=DIRECTION ( 'NONE',  ( 0.9980719161006958995, 0.06206811009758109871, -2.049912714059374948E-13 ) ) ;
#17774=DIRECTION ( 'NONE',  ( 1.526468026909999897E-13, 8.159623473500000156E-13, 1.000000000000000000 ) ) ;
#17781=DIRECTION ( 'NONE',  ( -8.523837997462170112E-12, 0.000000000000000000, 1.000000000000000000 ) ) ;
#17787=EDGE_CURVE ( 'NONE', #3534, #21497, #4380, .T. ) ;
#17789=VECTOR ( 'NONE', #14590, 1000.000000000000227 ) ;
#17810=ADVANCED_FACE ( 'NONE', ( #20805 ), #2262, .F. ) ;
#17817=ADVANCED_FACE ( 'NONE', ( #13184 ), #13532, .T. ) ;
#17824=EDGE_LOOP ( 'NONE', ( #1414, #13659, #14232, #6915 ) ) ;
#17836=AXIS2_PLACEMENT_3D ( 'NONE', #7489, #14754, #22021 ) ;
#17837=AXIS2_PLACEMENT_3D ( 'NONE', #16937, #7657, #773 ) ;
#17838=DIRECTION ( 'NONE',  ( 4.510774274160000731E-12, -1.321907670990000086E-13, 1.000000000000000000 ) ) ;
#17845=AXIS2_PLACEMENT_3D ( 'NONE', #7035, #21569, #3349 ) ;
#17852=VECTOR ( 'NONE', #16972, 1000.000000000000000 ) ;
#17856=LINE ( 'NONE', #5231, #5009 ) ;
#17859=AXIS2_PLACEMENT_3D ( 'NONE', #11519, #369, #7608 ) ;
#17874=VECTOR ( 'NONE', #2318, 1000.000000000000114 ) ;
#17879=CARTESIAN_POINT ( 'NONE',  ( 12.91075631260000023, -38.04527125359999928, -146.5552959529999839 ) ) ;
#17884=CARTESIAN_POINT ( 'NONE',  ( 16.29836742280000195, -22.74229684829999698, -143.5552959529999839 ) ) ;
#17891=FACE_OUTER_BOUND ( 'NONE', #1464, .T. ) ;
#17892=DIRECTION ( 'NONE',  ( 1.000000000000000000, 0.000000000000000000, -1.526556658859589738E-13 ) ) ;
#17893=DIRECTION ( 'NONE',  ( -4.510774274160000731E-12, 1.321907670990000086E-13, -1.000000000000000000 ) ) ;
#17897=ORIENTED_EDGE ( 'NONE', *, *, #16490, .T. ) ;
#17908=CARTESIAN_POINT ( 'NONE',  ( 12.91075631260000023, -38.04527125359999928, -146.5552959529999839 ) ) ;
#17915=ORIENTED_EDGE ( 'NONE', *, *, #2994, .T. ) ;
#17919=ORIENTED_EDGE ( 'NONE', *, *, #23077, .T. ) ;
#17924=DIRECTION ( 'NONE',  ( 1.000000000000000000, 0.000000000000000000, -4.429789868254374596E-12 ) ) ;
#17930=ORIENTED_EDGE ( 'NONE', *, *, #19734, .F. ) ;
#17936=ORIENTED_EDGE ( 'NONE', *, *, #6298, .F. ) ;
#17938=VECTOR ( 'NONE', #16456, 1000.000000000000227 ) ;
#17939=ADVANCED_FACE ( 'NONE', ( #15439 ), #6633, .T. ) ;
#17947=DIRECTION ( 'NONE',  ( 4.430318231639999944E-12, -6.100259101500000139E-13, 1.000000000000000000 ) ) ;
#17954=DIRECTION ( 'NONE',  ( -0.9913873220698726785, 0.1309625047069831461, -1.853446743629759619E-14 ) ) ;
#17958=AXIS2_PLACEMENT_3D ( 'NONE', #20356, #7954, #22022 ) ;
#17961=VERTEX_POINT ( 'NONE', #21281 ) ;
#17967=ADVANCED_FACE ( 'NONE', ( #2729 ), #6747, .T. ) ;
#17974=AXIS2_PLACEMENT_3D ( 'NONE', #9538, #13576, #4077 ) ;
#17975=FACE_OUTER_BOUND ( 'NONE', #3169, .T. ) ;
#17976=DIRECTION ( 'NONE',  ( 0.9985681355238719137, -0.05349466063429310358, -4.512926597569420539E-12 ) ) ;
#17978=CARTESIAN_POINT ( 'NONE',  ( 1.352544480119999948, -20.86379603889999856, -145.5552959529999839 ) ) ;
#17980=LINE ( 'NONE', #1691, #5750 ) ;
#17997=CARTESIAN_POINT ( 'NONE',  ( -0.6781431574100000859, -62.17334590100000469, -148.5552959529999839 ) ) ;
#18000=ORIENTED_EDGE ( 'NONE', *, *, #18880, .F. ) ;
#18016=LINE ( 'NONE', #5514, #8725 ) ;
#18029=EDGE_CURVE ( 'NONE', #10073, #1168, #1889, .T. ) ;
#18035=CARTESIAN_POINT ( 'NONE',  ( 16.74346552629999962, -18.31657829129999726, -148.0552959529999839 ) ) ;
#18039=ORIENTED_EDGE ( 'NONE', *, *, #11192, .T. ) ;
#18045=ORIENTED_EDGE ( 'NONE', *, *, #3134, .F. ) ;
#18048=CARTESIAN_POINT ( 'NONE',  ( 8.931951867280000457, -17.52729875919999714, -143.5552959529999839 ) ) ;
#18054=ORIENTED_EDGE ( 'NONE', *, *, #21676, .T. ) ;
#18058=ORIENTED_EDGE ( 'NONE', *, *, #16548, .T. ) ;
#18063=DIRECTION ( 'NONE',  ( 1.000000000000000000, 0.000000000000000000, -4.429789868254374596E-12 ) ) ;
#18067=ORIENTED_EDGE ( 'NONE', *, *, #13997, .F. ) ;
#18072=DIRECTION ( 'NONE',  ( -0.9954742291034676116, 0.09503188512734456195, 0.000000000000000000 ) ) ;
#18090=DIRECTION ( 'NONE',  ( 1.526468026909999897E-13, 8.159623473500000156E-13, 1.000000000000000000 ) ) ;
#18099=CARTESIAN_POINT ( 'NONE',  ( -9.334216945200001447, -17.19633444960000190, -145.5552959529999839 ) ) ;
#18114=ORIENTED_EDGE ( 'NONE', *, *, #21890, .T. ) ;
#18117=EDGE_CURVE ( 'NONE', #2929, #14604, #14603, .T. ) ;
#18120=EDGE_CURVE ( 'NONE', #13663, #2031, #3043, .T. ) ;
#18123=ORIENTED_EDGE ( 'NONE', *, *, #21262, .F. ) ;
#18125=DIRECTION ( 'NONE',  ( 0.000000000000000000, -1.000000000000000000, 3.568879590630000244E-13 ) ) ;
#18127=DIRECTION ( 'NONE',  ( 4.430318231639999944E-12, -6.100259101500000139E-13, 1.000000000000000000 ) ) ;
#18130=CARTESIAN_POINT ( 'NONE',  ( 23.41308733940000053, -15.43505800149999985, -148.0552959529999839 ) ) ;
#18133=DIRECTION ( 'NONE',  ( -0.09606172499277226828, -0.9953753789357124848, 8.289665250527615055E-13 ) ) ;
#18135=CARTESIAN_POINT ( 'NONE',  ( 16.87269471589999981, -31.91616505980000085, -144.5552959529999839 ) ) ;
#18144=CARTESIAN_POINT ( 'NONE',  ( 23.84377886109999878, -30.60602870049999780, -145.5552959529999839 ) ) ;
#18147=ORIENTED_EDGE ( 'NONE', *, *, #10682, .F. ) ;
#18154=CIRCLE ( 'NONE', #2577, 5.000000000000000000 ) ;
#18155=ORIENTED_EDGE ( 'NONE', *, *, #6046, .T. ) ;
#18158=VECTOR ( 'NONE', #703, 1000.000000000000227 ) ;
#18161=ORIENTED_EDGE ( 'NONE', *, *, #16233, .F. ) ;
#18172=VERTEX_POINT ( 'NONE', #19573 ) ;
#18178=CARTESIAN_POINT ( 'NONE',  ( 2.508811538190000245, -14.35090895149999923, -145.5552959529999839 ) ) ;
#18182=ORIENTED_EDGE ( 'NONE', *, *, #10866, .F. ) ;
#18184=LINE ( 'NONE', #16049, #14546 ) ;
#18189=VECTOR ( 'NONE', #19117, 1000.000000000000227 ) ;
#18195=LINE ( 'NONE', #22119, #10593 ) ;
#18210=CARTESIAN_POINT ( 'NONE',  ( 23.49999999970000175, -20.50000000000000000, -148.5552959529999839 ) ) ;
#18219=DIRECTION ( 'NONE',  ( 8.955190032050000935E-12, -9.104778821549999739E-13, 1.000000000000000000 ) ) ;
#18221=LINE ( 'NONE', #10939, #11338 ) ;
#18223=ORIENTED_EDGE ( 'NONE', *, *, #14577, .T. ) ;
#18244=EDGE_CURVE ( 'NONE', #6936, #16928, #8597, .T. ) ;
#18251=ORIENTED_EDGE ( 'NONE', *, *, #10866, .T. ) ;
#18271=UNCERTAINTY_MEASURE_WITH_UNIT (LENGTH_MEASURE( 1.000000000000000082E-05 ), #18596, 'distance_accuracy_value', 'NONE');
#18274=VERTEX_POINT ( 'NONE', #7308 ) ;
#18300=EDGE_LOOP ( 'NONE', ( #19997, #3778, #13960 ) ) ;
#18307=DIRECTION ( 'NONE',  ( -0.9919007982877544594, 0.1270149847699686418, 4.766005912188822159E-14 ) ) ;
#18313=VERTEX_POINT ( 'NONE', #20165 ) ;
#18316=VECTOR ( 'NONE', #627, 1000.000000000000114 ) ;
#18317=AXIS2_PLACEMENT_3D ( 'NONE', #17151, #9753, #15014 ) ;
#18319=ORIENTED_EDGE ( 'NONE', *, *, #2044, .F. ) ;
#18329=DIRECTION ( 'NONE',  ( 0.9834926989016489207, 0.1809478134909354718, -4.411697319228424767E-12 ) ) ;
#18330=CARTESIAN_POINT ( 'NONE',  ( 20.58976242830000203, -31.80400447969999789, -143.5552959529999839 ) ) ;
#18335=LINE ( 'NONE', #2395, #20535 ) ;
#18336=EDGE_CURVE ( 'NONE', #20005, #7769, #23373, .T. ) ;
#18337=DIRECTION ( 'NONE',  ( -0.04567108003750790929, 0.9989565318111732761, -8.081393722541401004E-13 ) ) ;
#18339=EDGE_CURVE ( 'NONE', #9011, #14876, #16205, .T. ) ;
#18340=LINE ( 'NONE', #5370, #7763 ) ;
#18344=VERTEX_POINT ( 'NONE', #9298 ) ;
#18347=ORIENTED_EDGE ( 'NONE', *, *, #21864, .T. ) ;
#18349=DIRECTION ( 'NONE',  ( -0.09606172499277228216, -0.9953753789357123738, 8.282644157540153068E-13 ) ) ;
#18351=CARTESIAN_POINT ( 'NONE',  ( 5.347956485829999274, -22.34165470570000167, -147.5552959529999839 ) ) ;
#18357=DIRECTION ( 'NONE',  ( -0.1739442350240419932, -0.9847555042252370550, 8.300754441162000146E-13 ) ) ;
#18360=EDGE_CURVE ( 'NONE', #6393, #7102, #1732, .T. ) ;
#18361=DIRECTION ( 'NONE',  ( 2.839308199620000013E-14, 3.568879590630000244E-13, 1.000000000000000000 ) ) ;
#18362=CARTESIAN_POINT ( 'NONE',  ( -9.434278515689999978, -18.41834002140000237, -147.5552959529999839 ) ) ;
#18364=DIRECTION ( 'NONE',  ( -0.09503188512734457583, -0.9954742291034677226, 2.970706163671393545E-13 ) ) ;
#18367=ORIENTED_EDGE ( 'NONE', *, *, #303, .T. ) ;
#18387=VERTEX_POINT ( 'NONE', #18135 ) ;
#18407=ORIENTED_EDGE ( 'NONE', *, *, #18623, .T. ) ;
#18411=EDGE_LOOP ( 'NONE', ( #22880, #12191 ) ) ;
#18416=LINE ( 'NONE', #569, #5316 ) ;
#18435=ORIENTED_EDGE ( 'NONE', *, *, #3502, .T. ) ;
#18436=DIRECTION ( 'NONE',  ( 0.1000233216789610108, 0.9949850929136109245, -3.588240815588595806E-13 ) ) ;
#18443=LINE ( 'NONE', #11282, #21633 ) ;
#18453=DIRECTION ( 'NONE',  ( -0.06298685227120542907, -0.9980143568310855251, 1.515824502950130739E-13 ) ) ;
#18454=ADVANCED_FACE ( 'NONE', ( #4298 ), #14889, .T. ) ;
#18455=DIRECTION ( 'NONE',  ( 1.527666881879999979E-13, 8.171241461240000022E-13, 1.000000000000000000 ) ) ;
#18458=AXIS2_PLACEMENT_3D ( 'NONE', #6167, #20685, #11618 ) ;
#18469=LINE ( 'NONE', #16683, #3960 ) ;
#18470=ORIENTED_EDGE ( 'NONE', *, *, #13374, .T. ) ;
#18473=AXIS2_PLACEMENT_3D ( 'NONE', #17879, #23113, #14187 ) ;
#18480=EDGE_CURVE ( 'NONE', #1486, #21613, #19632, .T. ) ;
#18523=DIRECTION ( 'NONE',  ( 1.000000000000000000, 0.000000000000000000, -1.498801083243961330E-13 ) ) ;
#18524=DIRECTION ( 'NONE',  ( -2.842170943040000002E-14, -3.570477247189999985E-13, -1.000000000000000000 ) ) ;
#18531=EDGE_CURVE ( 'NONE', #13091, #21066, #5722, .T. ) ;
#18533=DIRECTION ( 'NONE',  ( -0.9892101392001054760, 0.1465035852930155480, 4.471739159800472250E-12 ) ) ;
#18541=ORIENTED_EDGE ( 'NONE', *, *, #4351, .F. ) ;
#18546=DIRECTION ( 'NONE',  ( -1.527666881879999979E-13, -8.171241461240000022E-13, -1.000000000000000000 ) ) ;
#18554=AXIS2_PLACEMENT_3D ( 'NONE', #12239, #2978, #19034 ) ;
#18555=DIRECTION ( 'NONE',  ( -0.1435602414469281940, -0.9896415801065048257, 3.836930773098079160E-13 ) ) ;
#18559=CARTESIAN_POINT ( 'NONE',  ( 1.713198289069999936, -17.44292009260000142, -147.5552959529999839 ) ) ;
#18567=EDGE_CURVE ( 'NONE', #13091, #12006, #7079, .T. ) ;
#18576=CARTESIAN_POINT ( 'NONE',  ( 24.36715301250000110, -30.57462384669999977, -147.5552959529999839 ) ) ;
#18587=CIRCLE ( 'NONE', #17845, 6.000000000000001776 ) ;
#18591=DIRECTION ( 'NONE',  ( -0.9938526945756316344, 0.1107105301439589573, 6.178155812097707047E-14 ) ) ;
#18592=VECTOR ( 'NONE', #19658, 1000.000000000000000 ) ;
#18594=EDGE_LOOP ( 'NONE', ( #2585, #17437, #21133 ) ) ;
#18595=CIRCLE ( 'NONE', #11351, 5.000000000000000000 ) ;
#18596=( LENGTH_UNIT ( ) NAMED_UNIT ( * ) SI_UNIT ( .MILLI., .METRE. ) );
#18605=DIRECTION ( 'NONE',  ( -0.1146332952500066227, -0.9934078757590583120, -9.947598300640582187E-14 ) ) ;
#18609=VERTEX_POINT ( 'NONE', #20955 ) ;
#18616=VECTOR ( 'NONE', #8304, 1000.000000000000000 ) ;
#18617=ORIENTED_EDGE ( 'NONE', *, *, #12858, .F. ) ;
#18623=EDGE_CURVE ( 'NONE', #11516, #5773, #6541, .T. ) ;
#18631=AXIS2_PLACEMENT_3D ( 'NONE', #13853, #22658, #6589 ) ;
#18632=DIRECTION ( 'NONE',  ( -8.955503005839999404E-12, 9.112710586119999183E-13, -1.000000000000000000 ) ) ;
#18638=ORIENTED_EDGE ( 'NONE', *, *, #10917, .F. ) ;
#18646=CIRCLE ( 'NONE', #6095, 5.000000000000000000 ) ;
#18669=VERTEX_POINT ( 'NONE', #6302 ) ;
#18670=CARTESIAN_POINT ( 'NONE',  ( 1.561837858109999866, -18.84848306830000197, -143.5552959529999839 ) ) ;
#18675=LINE ( 'NONE', #2387, #16793 ) ;
#18677=DIRECTION ( 'NONE',  ( -2.842170943040000002E-14, -3.552713678800000097E-13, -1.000000000000000000 ) ) ;
#18684=DIRECTION ( 'NONE',  ( 1.000000000000000000, 0.000000000000000000, -8.955190032050000935E-12 ) ) ;
#18686=VECTOR ( 'NONE', #22511, 1000.000000000000114 ) ;
#18690=VERTEX_POINT ( 'NONE', #5470 ) ;
#18693=ORIENTED_EDGE ( 'NONE', *, *, #20641, .F. ) ;
#18696=ORIENTED_EDGE ( 'NONE', *, *, #3286, .F. ) ;
#18709=CARTESIAN_POINT ( 'NONE',  ( 16.64676602990000021, -18.64223989710000140, -143.5552959529999839 ) ) ;
#18718=PLANE ( 'NONE',  #4716 ) ;
#18732=LINE ( 'NONE', #10013, #7791 ) ;
#18737=ORIENTED_EDGE ( 'NONE', *, *, #20103, .T. ) ;
#18745=DIRECTION ( 'NONE',  ( -0.09606172499277226828, -0.9953753789357124848, 8.268372250837614805E-13 ) ) ;
#18752=EDGE_CURVE ( 'NONE', #20549, #12827, #21661, .T. ) ;
#18753=DIRECTION ( 'NONE',  ( 1.000000000000000000, 0.000000000000000000, -4.430318231639999944E-12 ) ) ;
#18754=ORIENTED_EDGE ( 'NONE', *, *, #3134, .T. ) ;
#18766=DIRECTION ( 'NONE',  ( 1.526468026909999897E-13, 8.159623473500000156E-13, 1.000000000000000000 ) ) ;
#18767=LINE ( 'NONE', #12938, #4506 ) ;
#18779=DIRECTION ( 'NONE',  ( 1.000000000000000000, 0.000000000000000000, -4.430318231639999944E-12 ) ) ;
#18785=CARTESIAN_POINT ( 'NONE',  ( 2.531727043930000143, -11.80034048859999807, -148.0552959529999839 ) ) ;
#18795=DIRECTION ( 'NONE',  ( -0.9800948705872890576, 0.1985297072190584933, -1.238441759210365047E-14 ) ) ;
#18801=EDGE_CURVE ( 'NONE', #2700, #14669, #16060, .T. ) ;
#18807=LINE ( 'NONE', #6544, #6446 ) ;
#18811=CARTESIAN_POINT ( 'NONE',  ( 17.58326321919999558, -18.99156222550000095, -146.5552959529999839 ) ) ;
#18820=LINE ( 'NONE', #2769, #23269 ) ;
#18827=EDGE_CURVE ( 'NONE', #473, #2813, #9253, .T. ) ;
#18829=AXIS2_PLACEMENT_3D ( 'NONE', #18576, #15362, #5842 ) ;
#18832=ORIENTED_EDGE ( 'NONE', *, *, #1543, .F. ) ;
#18847=VECTOR ( 'NONE', #3739, 1000.000000000000000 ) ;
#18863=CARTESIAN_POINT ( 'NONE',  ( 22.36721601470000209, -21.34320095609999868, -147.5552959529999839 ) ) ;
#18867=CARTESIAN_POINT ( 'NONE',  ( -9.876524491812205042, -22.81279121395682807, -144.5552959529502743 ) ) ;
#18868=ORIENTED_EDGE ( 'NONE', *, *, #23137, .T. ) ;
#18871=FACE_OUTER_BOUND ( 'NONE', #302, .T. ) ;
#18876=VECTOR ( 'NONE', #2032, 1000.000000000000227 ) ;
#18880=EDGE_CURVE ( 'NONE', #20938, #22607, #13065, .T. ) ;
#18884=EDGE_CURVE ( 'NONE', #13434, #11590, #12950, .T. ) ;
#18885=DIRECTION ( 'NONE',  ( 0.000000000000000000, -1.000000000000000000, 8.159623473500000156E-13 ) ) ;
#18891=AXIS2_PLACEMENT_3D ( 'NONE', #7507, #9520, #9631 ) ;
#18894=ORIENTED_EDGE ( 'NONE', *, *, #14085, .T. ) ;
#18907=DIRECTION ( 'NONE',  ( -1.263593756457750072E-14, 0.000000000000000000, 1.000000000000000000 ) ) ;
#18926=LINE ( 'NONE', #13098, #4392 ) ;
#18928=PLANE ( 'NONE',  #5996 ) ;
#18941=EDGE_CURVE ( 'NONE', #13141, #5742, #125, .T. ) ;
#18944=AXIS2_PLACEMENT_3D ( 'NONE', #13928, #2993, #15365 ) ;
#18953=LINE ( 'NONE', #9892, #21251 ) ;
#18954=CARTESIAN_POINT ( 'NONE',  ( 23.63070326403130039, -30.71011948576827066, -147.5552959530019166 ) ) ;
#18971=LINE ( 'NONE', #1143, #9486 ) ;
#18976=VECTOR ( 'NONE', #23109, 1000.000000000000000 ) ;
#18977=DIRECTION ( 'NONE',  ( 8.956391184260000029E-12, -9.094947017729999296E-13, 1.000000000000000000 ) ) ;
#18982=DIRECTION ( 'NONE',  ( 2.842170943040000002E-14, 3.570477247189999985E-13, 1.000000000000000000 ) ) ;
#18984=VECTOR ( 'NONE', #6530, 999.9999999999998863 ) ;
#18985=AXIS2_PLACEMENT_3D ( 'NONE', #6662, #5361, #10693 ) ;
#18989=DIRECTION ( 'NONE',  ( -2.839308199620000013E-14, -3.568879590630000244E-13, -1.000000000000000000 ) ) ;
#18996=ORIENTED_EDGE ( 'NONE', *, *, #23539, .T. ) ;
#19006=CARTESIAN_POINT ( 'NONE',  ( 4.128836048080000154, -25.17057797350000214, -147.5552959529999839 ) ) ;
#19012=DIRECTION ( 'NONE',  ( 8.954614827420000395E-12, -9.112710586119999183E-13, 1.000000000000000000 ) ) ;
#19018=VERTEX_POINT ( 'NONE', #6715 ) ;
#19019=LINE ( 'NONE', #17346, #7222 ) ;
#19023=ADVANCED_FACE ( 'NONE', ( #23028 ), #11825, .T. ) ;
#19026=CARTESIAN_POINT ( 'NONE',  ( 27.02097087391203800, -17.55867353012727250, -143.5552959530038208 ) ) ;
#19029=LINE ( 'NONE', #10205, #865 ) ;
#19030=VERTEX_POINT ( 'NONE', #10395 ) ;
#19032=EDGE_LOOP ( 'NONE', ( #15347, #10045, #23363 ) ) ;
#19034=DIRECTION ( 'NONE',  ( -0.9919007982877544594, 0.1270149847699686418, 0.000000000000000000 ) ) ;
#19040=CARTESIAN_POINT ( 'NONE',  ( -9.812199629310001114, -24.40642616239999896, -146.5552959529999839 ) ) ;
#19048=LINE ( 'NONE', #15601, #18686 ) ;
#19060=ORIENTED_EDGE ( 'NONE', *, *, #4687, .F. ) ;
#19065=ADVANCED_FACE ( 'NONE', ( #6835 ), #14102, .T. ) ;
#19071=ORIENTED_EDGE ( 'NONE', *, *, #16949, .T. ) ;
#19072=AXIS2_PLACEMENT_3D ( 'NONE', #19800, #18361, #16341 ) ;
#19117=DIRECTION ( 'NONE',  ( -0.1146332952500066227, -0.9934078757590583120, -9.947598300640582187E-14 ) ) ;
#19119=LINE ( 'NONE', #19006, #1512 ) ;
#19127=EDGE_CURVE ( 'NONE', #9406, #18690, #19688, .T. ) ;
#19136=FACE_OUTER_BOUND ( 'NONE', #17635, .T. ) ;
#19144=EDGE_LOOP ( 'NONE', ( #12739, #10042, #3516, #13803, #2809 ) ) ;
#19146=DIRECTION ( 'NONE',  ( -0.9968185442904002880, 0.07970438983373201447, 8.712538262633493651E-14 ) ) ;
#19153=CIRCLE ( 'NONE', #15744, 6.000000000000001776 ) ;
#19154=ADVANCED_FACE ( 'NONE', ( #20047 ), #66, .F. ) ;
#19155=EDGE_LOOP ( 'NONE', ( #20780, #23015, #5916, #23070, #215 ) ) ;
#19157=DIRECTION ( 'NONE',  ( 7.389987738588579788E-14, 0.000000000000000000, 1.000000000000000000 ) ) ;
#19159=CARTESIAN_POINT ( 'NONE',  ( -9.334216945200001447, -17.19633444960000190, -146.5552959529999839 ) ) ;
#19163=CARTESIAN_POINT ( 'NONE',  ( -9.873006318519999880, -23.84776512999999909, -142.5552959529999839 ) ) ;
#19164=CARTESIAN_POINT ( 'NONE',  ( 17.21087225569999646, -22.66053313549999970, -145.0552959529999839 ) ) ;
#19169=VECTOR ( 'NONE', #3344, 1000.000000000000000 ) ;
#19170=DIRECTION ( 'NONE',  ( -0.9954742291034677226, 0.09503188512734457583, 4.502513436702118395E-12 ) ) ;
#19171=DIRECTION ( 'NONE',  ( 1.000000000000000000, 0.000000000000000000, -4.510281037539696830E-12 ) ) ;
#19172=CARTESIAN_POINT ( 'NONE',  ( 23.50000000000000000, -20.50000000000000000, -142.5552959529999839 ) ) ;
#19187=CARTESIAN_POINT ( 'NONE',  ( 16.16922456049999823, -22.27514461170000004, -147.5552959529999839 ) ) ;
#19198=VERTEX_POINT ( 'NONE', #14456 ) ;
#19202=ORIENTED_EDGE ( 'NONE', *, *, #2222, .F. ) ;
#19219=DIRECTION ( 'NONE',  ( 1.000000000000000000, 0.000000000000000000, -2.854859206178974232E-14 ) ) ;
#19220=EDGE_LOOP ( 'NONE', ( #13437, #8523, #22518, #13566 ) ) ;
#19222=ORIENTED_EDGE ( 'NONE', *, *, #12301, .T. ) ;
#19232=ORIENTED_EDGE ( 'NONE', *, *, #19, .T. ) ;
#19236=VECTOR ( 'NONE', #3166, 1000.000000000000114 ) ;
#19243=ORIENTED_EDGE ( 'NONE', *, *, #22294, .F. ) ;
#19250=VECTOR ( 'NONE', #14682, 1000.000000000000227 ) ;
#19256=VERTEX_POINT ( 'NONE', #18954 ) ;
#19268=AXIS2_PLACEMENT_3D ( 'NONE', #11675, #17286, #21103 ) ;
#19273=EDGE_CURVE ( 'NONE', #760, #7372, #7530, .T. ) ;
#19291=DIRECTION ( 'NONE',  ( 1.000000000000000000, 0.000000000000000000, -1.527536832333223921E-13 ) ) ;
#19294=EDGE_CURVE ( 'NONE', #12291, #14669, #20746, .T. ) ;
#19306=AXIS2_PLACEMENT_3D ( 'NONE', #22798, #11588, #6493 ) ;
#19309=ORIENTED_EDGE ( 'NONE', *, *, #10243, .F. ) ;
#19311=DIRECTION ( 'NONE',  ( 0.9834926989016489207, 0.1809478134909354718, -4.411697319228424767E-12 ) ) ;
#19313=CARTESIAN_POINT ( 'NONE',  ( 20.31210873290000052, -31.32069079449999904, -147.5552959529999839 ) ) ;
#19353=ORIENTED_EDGE ( 'NONE', *, *, #6208, .T. ) ;
#19354=CARTESIAN_POINT ( 'NONE',  ( 8.995627988029999855, -17.23072307649999857, -145.5552959529999839 ) ) ;
#19359=AXIS2_PLACEMENT_3D ( 'NONE', #22822, #22945, #23055 ) ;
#19361=ORIENTED_EDGE ( 'NONE', *, *, #16022, .T. ) ;
#19363=DIRECTION ( 'NONE',  ( 1.526468026911395108E-13, 8.159623473499890094E-13, 1.000000000000000000 ) ) ;
#19373=ORIENTED_EDGE ( 'NONE', *, *, #7906, .F. ) ;
#19376=VERTEX_POINT ( 'NONE', #20634 ) ;
#19390=CIRCLE ( 'NONE', #776, 8.176568160360000448 ) ;
#19391=FACE_OUTER_BOUND ( 'NONE', #10023, .T. ) ;
#19393=DIRECTION ( 'NONE',  ( -0.9954742291034677226, 0.09503188512734457583, 4.502513436702118395E-12 ) ) ;
#19399=VECTOR ( 'NONE', #13773, 1000.000000000000000 ) ;
#19404=CARTESIAN_POINT ( 'NONE',  ( -6.599319970649999867, -19.98386714700000155, -145.5552959529999839 ) ) ;
#19410=CARTESIAN_POINT ( 'NONE',  ( -2.203055323360000095, -15.74846988260000025, -142.5552959529999839 ) ) ;
#19416=DIRECTION ( 'NONE',  ( -2.839308199620000013E-14, -3.568879590630000244E-13, -1.000000000000000000 ) ) ;
#19423=ORIENTED_EDGE ( 'NONE', *, *, #9952, .F. ) ;
#19438=CARTESIAN_POINT ( 'NONE',  ( 16.74346552629999962, -18.31657829129999726, -147.5552959529999839 ) ) ;
#19441=LINE ( 'NONE', #6811, #7142 ) ;
#19442=DIRECTION ( 'NONE',  ( 0.1985297072190585210, 0.9800948705872890576, -8.292396948122451413E-13 ) ) ;
#19444=ORIENTED_EDGE ( 'NONE', *, *, #956, .T. ) ;
#19446=SURFACE_STYLE_FILL_AREA ( #21112 ) ;
#19447=VERTEX_POINT ( 'NONE', #3837 ) ;
#19454=VECTOR ( 'NONE', #19442, 1000.000000000000114 ) ;
#19460=DIRECTION ( 'NONE',  ( 4.511946372079999833E-12, -1.314504061159999897E-13, 1.000000000000000000 ) ) ;
#19462=LINE ( 'NONE', #410, #23391 ) ;
#19466=LINE ( 'NONE', #10747, #22283 ) ;
#19472=AXIS2_PLACEMENT_3D ( 'NONE', #20944, #19146, #13670 ) ;
#19478=LINE ( 'NONE', #1515, #17547 ) ;
#19479=ORIENTED_EDGE ( 'NONE', *, *, #10482, .T. ) ;
#19484=DIRECTION ( 'NONE',  ( 0.002160933882609249439, 0.9999976651796518290, 8.911241827866908793E-13 ) ) ;
#19493=VERTEX_POINT ( 'NONE', #2063 ) ;
#19501=ORIENTED_EDGE ( 'NONE', *, *, #6960, .T. ) ;
#19509=DIRECTION ( 'NONE',  ( -0.9892101392001054760, 0.1465035852930155480, 4.472400123700476920E-12 ) ) ;
#19515=ADVANCED_FACE ( 'NONE', ( #4188 ), #265, .F. ) ;
#19517=ADVANCED_FACE ( 'NONE', ( #11299 ), #13211, .F. ) ;
#19526=LINE ( 'NONE', #8665, #12912 ) ;
#19534=CARTESIAN_POINT ( 'NONE',  ( -8.594304764359998572, -10.75357442870000035, -145.5552959529999839 ) ) ;
#19537=EDGE_CURVE ( 'NONE', #712, #19545, #5841, .T. ) ;
#19538=ORIENTED_EDGE ( 'NONE', *, *, #18801, .F. ) ;
#19544=CARTESIAN_POINT ( 'NONE',  ( 16.65421564080000039, -18.61497348660000029, -145.5552959529999839 ) ) ;
#19545=VERTEX_POINT ( 'NONE', #16905 ) ;
#19547=CARTESIAN_POINT ( 'NONE',  ( 6.477506801250000557, -13.91317765220000169, -147.5552959529999839 ) ) ;
#19564=ORIENTED_EDGE ( 'NONE', *, *, #6593, .T. ) ;
#19566=CARTESIAN_POINT ( 'NONE',  ( -6.270646159103367978, -16.71437421844448323, -146.5552959529736654 ) ) ;
#19573=CARTESIAN_POINT ( 'NONE',  ( 16.33424841169999908, -31.58611763329999889, -147.5552959529999839 ) ) ;
#19576=DIRECTION ( 'NONE',  ( -0.9840552701943220404, 0.1778629393740580045, -3.541738516501160129E-14 ) ) ;
#19582=ORIENTED_EDGE ( 'NONE', *, *, #17136, .F. ) ;
#19585=ORIENTED_EDGE ( 'NONE', *, *, #13310, .F. ) ;
#19586=AXIS2_PLACEMENT_3D ( 'NONE', #15767, #8726, #10628 ) ;
#19591=VERTEX_POINT ( 'NONE', #17261 ) ;
#19598=ORIENTED_EDGE ( 'NONE', *, *, #8404, .T. ) ;
#19602=CARTESIAN_POINT ( 'NONE',  ( -5.758148842630000708, -13.22138763369999914, -147.5552959529999839 ) ) ;
#19608=CARTESIAN_POINT ( 'NONE',  ( 5.276897646260000130, -21.39828525539999760, -144.5552959529999839 ) ) ;
#19614=LINE ( 'NONE', #21409, #4568 ) ;
#19624=CARTESIAN_POINT ( 'NONE',  ( 2.170391987449999505, -12.72823260819999902, -146.5552959529999839 ) ) ;
#19632=CIRCLE ( 'NONE', #23051, 5.999999999999998224 ) ;
#19635=LINE ( 'NONE', #1571, #3652 ) ;
#19636=DIRECTION ( 'NONE',  ( -0.9919007982877544594, 0.1270149847699686418, 4.677746543438841512E-14 ) ) ;
#19637=DIRECTION ( 'NONE',  ( 0.06298685227120542907, 0.9980143568310855251, -1.492139745100128694E-13 ) ) ;
#19639=CARTESIAN_POINT ( 'NONE',  ( 2.139623390130000136, -12.81320239329999922, -144.5552959529999839 ) ) ;
#19649=AXIS2_PLACEMENT_3D ( 'NONE', #12771, #20045, #14681 ) ;
#19650=ORIENTED_EDGE ( 'NONE', *, *, #23539, .F. ) ;
#19655=PRODUCT ( 'Lock Tumblers', 'Lock Tumblers', '', ( #3784 ) ) ;
#19656=CARTESIAN_POINT ( 'NONE',  ( -6.601136089949999786, -20.10368962670000315, -143.5552959529999839 ) ) ;
#19658=DIRECTION ( 'NONE',  ( 8.954614827420000395E-12, -9.094947017729999296E-13, 1.000000000000000000 ) ) ;
#19659=LINE ( 'NONE', #19547, #11996 ) ;
#19660=DIRECTION ( 'NONE',  ( -0.09606172499277226828, -0.9953753789357124848, 8.268133652477615271E-13 ) ) ;
#19676=CARTESIAN_POINT ( 'NONE',  ( 21.39890631740000160, -21.26106171180000359, -144.5552959529999839 ) ) ;
#19677=CARTESIAN_POINT ( 'NONE',  ( 24.87050155979999744, -26.86223000240000047, -145.5552959529999839 ) ) ;
#19679=CARTESIAN_POINT ( 'NONE',  ( -9.347107914279998653, -17.32706600430000066, -143.5552959529999839 ) ) ;
#19686=FACE_OUTER_BOUND ( 'NONE', #2291, .T. ) ;
#19688=LINE ( 'NONE', #21952, #19250 ) ;
#19689=PLANE ( 'NONE',  #961 ) ;
#19690=ADVANCED_FACE ( 'NONE', ( #20714 ), #12127, .T. ) ;
#19699=ORIENTED_EDGE ( 'NONE', *, *, #13973, .T. ) ;
#19705=VERTEX_POINT ( 'NONE', #8090 ) ;
#19712=EDGE_LOOP ( 'NONE', ( #20870, #16389, #10107, #4016, #10967 ) ) ;
#19718=LINE ( 'NONE', #10887, #7216 ) ;
#19723=EDGE_CURVE ( 'NONE', #7689, #4619, #3329, .T. ) ;
#19725=ORIENTED_EDGE ( 'NONE', *, *, #10934, .F. ) ;
#19734=EDGE_CURVE ( 'NONE', #19705, #2700, #14524, .T. ) ;
#19735=CARTESIAN_POINT ( 'NONE',  ( 2.508811538190000245, -14.35090895149999923, -145.5552959529999839 ) ) ;
#19736=VERTEX_POINT ( 'NONE', #14394 ) ;
#19738=AXIS2_PLACEMENT_3D ( 'NONE', #19544, #15842, #22885 ) ;
#19761=CARTESIAN_POINT ( 'NONE',  ( -2.100773033209999863, -15.22510554480000167, -146.5552959529999839 ) ) ;
#19763=LINE ( 'NONE', #133, #22432 ) ;
#19773=FACE_OUTER_BOUND ( 'NONE', #2775, .T. ) ;
#19779=CIRCLE ( 'NONE', #22418, 14.99999999999999822 ) ;
#19780=VECTOR ( 'NONE', #22904, 1000.000000000000000 ) ;
#19787=DIRECTION ( 'NONE',  ( 1.000000000000000000, 0.000000000000000000, -4.511206223393553012E-12 ) ) ;
#19796=VECTOR ( 'NONE', #22012, 1000.000000000000000 ) ;
#19800=CARTESIAN_POINT ( 'NONE',  ( -9.334216945200001447, -17.19633444960000190, -145.5552959529999839 ) ) ;
#19804=DIRECTION ( 'NONE',  ( -0.9753087663813413410, 0.2208456705930775810, 0.000000000000000000 ) ) ;
#19805=DIRECTION ( 'NONE',  ( -0.1000233216789610108, -0.9949850929136109245, 3.576398436658600095E-13 ) ) ;
#19808=FACE_OUTER_BOUND ( 'NONE', #18594, .T. ) ;
#19810=AXIS2_PLACEMENT_3D ( 'NONE', #9684, #558, #21349 ) ;
#19818=CARTESIAN_POINT ( 'NONE',  ( -9.334216945200001447, -17.19633444960000190, -146.5552959529999839 ) ) ;
#19833=DIRECTION ( 'NONE',  ( 0.1720749717299729364, 0.9850838563818457017, -6.484322019408987829E-13 ) ) ;
#19836=EDGE_CURVE ( 'NONE', #18609, #22206, #7710, .T. ) ;
#19837=ORIENTED_EDGE ( 'NONE', *, *, #1689, .F. ) ;
#19840=DIRECTION ( 'NONE',  ( 2.839308199620000013E-14, 3.568879590630000244E-13, 1.000000000000000000 ) ) ;
#19842=EDGE_CURVE ( 'NONE', #21873, #6393, #14977, .T. ) ;
#19843=ORIENTED_EDGE ( 'NONE', *, *, #11522, .T. ) ;
#19846=DIRECTION ( 'NONE',  ( 2.839308199593065147E-14, 3.568879590624614785E-13, 1.000000000000000000 ) ) ;
#19851=EDGE_LOOP ( 'NONE', ( #23338, #19353 ) ) ;
#19861=DIRECTION ( 'NONE',  ( 0.1824094679249879947, 0.9832226533249336375, -8.292396948119437334E-13 ) ) ;
#19871=ORIENTED_EDGE ( 'NONE', *, *, #6911, .T. ) ;
#19880=VECTOR ( 'NONE', #1106, 1000.000000000000114 ) ;
#19885=ORIENTED_EDGE ( 'NONE', *, *, #513, .F. ) ;
#19897=CARTESIAN_POINT ( 'NONE',  ( 1.759100530420000030, -16.38142836440000139, -142.5552959529999839 ) ) ;
#19915=DIRECTION ( 'NONE',  ( -0.1577507813030449846, -0.9874789572432817186, 8.298258002992369366E-13 ) ) ;
#19921=DIRECTION ( 'NONE',  ( 8.955190032050000935E-12, -9.104778821549999739E-13, 1.000000000000000000 ) ) ;
#19929=CARTESIAN_POINT ( 'NONE',  ( 16.64676602990000021, -18.64223989710000140, -144.5552959529999839 ) ) ;
#19932=ORIENTED_EDGE ( 'NONE', *, *, #12946, .T. ) ;
#19938=DIRECTION ( 'NONE',  ( 1.000000000000000000, 0.000000000000000000, -1.498801083243961330E-13 ) ) ;
#19956=AXIS2_PLACEMENT_3D ( 'NONE', #15708, #17613, #22970 ) ;
#19957=FACE_OUTER_BOUND ( 'NONE', #1066, .T. ) ;
#19959=ORIENTED_EDGE ( 'NONE', *, *, #15505, .F. ) ;
#19961=VERTEX_POINT ( 'NONE', #6632 ) ;
#19965=ORIENTED_EDGE ( 'NONE', *, *, #8137, .F. ) ;
#19972=CARTESIAN_POINT ( 'NONE',  ( 8.890149109412865513, -17.38667989274045311, -145.5552959530314467 ) ) ;
#19976=DIRECTION ( 'NONE',  ( 0.9985681355238719137, -0.05349466063429310358, -4.512926597569420539E-12 ) ) ;
#19979=CARTESIAN_POINT ( 'NONE',  ( -9.394779979509999990, -17.86685386420000299, -143.5552959529999839 ) ) ;
#19982=CARTESIAN_POINT ( 'NONE',  ( 5.276897646250000129, -21.39828525539999760, -145.5552959529999839 ) ) ;
#19983=LINE ( 'NONE', #9137, #2484 ) ;
#19988=LINE ( 'NONE', #10691, #13906 ) ;
#19994=DIRECTION ( 'NONE',  ( 1.000000000000000000, 0.000000000000000000, -8.955799065309598247E-12 ) ) ;
#19997=ORIENTED_EDGE ( 'NONE', *, *, #3286, .T. ) ;
#20005=VERTEX_POINT ( 'NONE', #13415 ) ;
#20007=DIRECTION ( 'NONE',  ( -0.06298685227120542907, -0.9980143568310855251, 1.515824502950130739E-13 ) ) ;
#20010=VECTOR ( 'NONE', #8955, 1000.000000000000000 ) ;
#20012=EDGE_CURVE ( 'NONE', #22329, #11927, #21047, .T. ) ;
#20026=ORIENTED_EDGE ( 'NONE', *, *, #7473, .T. ) ;
#20030=VECTOR ( 'NONE', #18982, 1000.000000000000000 ) ;
#20033=DIRECTION ( 'NONE',  ( 1.000000000000000000, 0.000000000000000000, -4.510281037539699253E-12 ) ) ;
#20045=DIRECTION ( 'NONE',  ( 4.510774274160000731E-12, -1.321907670990000086E-13, 1.000000000000000000 ) ) ;
#20047=FACE_OUTER_BOUND ( 'NONE', #21802, .T. ) ;
#20056=CARTESIAN_POINT ( 'NONE',  ( 2.508811538200000246, -14.35090895149999923, -144.5552959529999839 ) ) ;
#20065=DIRECTION ( 'NONE',  ( -0.9954742291034677226, 0.09503188512734457583, 4.502513436702118395E-12 ) ) ;
#20071=ADVANCED_FACE ( 'NONE', ( #19957 ), #12330, .T. ) ;
#20072=AXIS2_PLACEMENT_3D ( 'NONE', #1953, #15008, #5959 ) ;
#20094=CARTESIAN_POINT ( 'NONE',  ( -9.434278515689999978, -18.41834002140000237, -147.5552959529999839 ) ) ;
#20102=DIRECTION ( 'NONE',  ( -8.954614827420000395E-12, 9.094947017729999296E-13, -1.000000000000000000 ) ) ;
#20103=EDGE_CURVE ( 'NONE', #404, #2894, #17590, .T. ) ;
#20110=AXIS2_PLACEMENT_3D ( 'NONE', #10495, #7307, #16354 ) ;
#20115=CIRCLE ( 'NONE', #2633, 15.00000000000000000 ) ;
#20120=CARTESIAN_POINT ( 'NONE',  ( -4.192924954330000453, -28.60725908990000121, -146.0552959529999839 ) ) ;
#20124=LINE ( 'NONE', #8805, #14235 ) ;
#20127=PLANE ( 'NONE',  #21993 ) ;
#20130=EDGE_CURVE ( 'NONE', #19030, #19493, #14755, .T. ) ;
#20138=DIRECTION ( 'NONE',  ( 1.000000000000000000, 0.000000000000000000, -8.955534726494208689E-12 ) ) ;
#20153=CARTESIAN_POINT ( 'NONE',  ( -4.946601369560000627, -23.77962690289999870, -143.5552959529999839 ) ) ;
#20155=VECTOR ( 'NONE', #12526, 1000.000000000000227 ) ;
#20165=CARTESIAN_POINT ( 'NONE',  ( 23.21181482501885185, -23.48612613683581785, -148.5552959530001260 ) ) ;
#20175=AXIS2_PLACEMENT_3D ( 'NONE', #16025, #23286, #6978 ) ;
#20177=ORIENTED_EDGE ( 'NONE', *, *, #13614, .F. ) ;
#20179=EDGE_LOOP ( 'NONE', ( #13848, #1913, #19479, #17054, #2173 ) ) ;
#20184=DIRECTION ( 'NONE',  ( 1.526468026909999897E-13, 8.159623473500000156E-13, 1.000000000000000000 ) ) ;
#20196=CARTESIAN_POINT ( 'NONE',  ( 8.931951867280000457, -17.52729875919999714, -142.5552959529999839 ) ) ;
#20200=ORIENTED_EDGE ( 'NONE', *, *, #1490, .F. ) ;
#20210=ORIENTED_EDGE ( 'NONE', *, *, #3052, .T. ) ;
#20225=PLANE ( 'NONE',  #11353 ) ;
#20252=ORIENTED_EDGE ( 'NONE', *, *, #1211, .F. ) ;
#20255=CIRCLE ( 'NONE', #17195, 6.000000000000001776 ) ;
#20268=DIRECTION ( 'NONE',  ( 1.526468026909999897E-13, 8.159623473500000156E-13, 1.000000000000000000 ) ) ;
#20270=FACE_OUTER_BOUND ( 'NONE', #15236, .T. ) ;
#20286=VECTOR ( 'NONE', #3755, 1000.000000000000000 ) ;
#20305=VECTOR ( 'NONE', #9643, 1000.000000000000000 ) ;
#20309=ORIENTED_EDGE ( 'NONE', *, *, #16233, .T. ) ;
#20313=EDGE_LOOP ( 'NONE', ( #401, #12266, #18223, #1598, #1876 ) ) ;
#20315=EDGE_CURVE ( 'NONE', #13630, #7372, #17197, .T. ) ;
#20324=EDGE_CURVE ( 'NONE', #3534, #7769, #4240, .T. ) ;
#20330=CARTESIAN_POINT ( 'NONE',  ( -4.872173186980353066, -28.66560015775754167, -146.5552959530116652 ) ) ;
#20334=DIRECTION ( 'NONE',  ( -2.909421006506540042E-11, 0.000000000000000000, -1.000000000000000000 ) ) ;
#20341=EDGE_LOOP ( 'NONE', ( #4394, #5538, #18058 ) ) ;
#20356=CARTESIAN_POINT ( 'NONE',  ( -9.157754307290000284, -15.75963164970000108, -147.5552959529999839 ) ) ;
#20359=PLANE ( 'NONE',  #7546 ) ;
#20361=VERTEX_POINT ( 'NONE', #16962 ) ;
#20362=ORIENTED_EDGE ( 'NONE', *, *, #21676, .F. ) ;
#20364=CARTESIAN_POINT ( 'NONE',  ( 1.364575185789999923, -21.31553777220000256, -143.0552959529999839 ) ) ;
#20365=LINE ( 'NONE', #18351, #5219 ) ;
#20367=ORIENTED_EDGE ( 'NONE', *, *, #4657, .F. ) ;
#20371=EDGE_CURVE ( 'NONE', #712, #2852, #672, .T. ) ;
#20376=ADVANCED_FACE ( 'NONE', ( #20658 ), #22562, .T. ) ;
#20379=DIRECTION ( 'NONE',  ( 1.000000000000000000, 0.000000000000000000, -4.510774274160000731E-12 ) ) ;
#20383=CARTESIAN_POINT ( 'NONE',  ( 22.40884248670000289, -21.39641658300000060, -144.5552959529999839 ) ) ;
#20397=LINE ( 'NONE', #12775, #14752 ) ;
#20405=DIRECTION ( 'NONE',  ( -0.09606172499277226828, -0.9953753789357124848, 8.265980492677616040E-13 ) ) ;
#20409=ADVANCED_FACE ( 'NONE', ( #17081 ), #4707, .F. ) ;
#20411=EDGE_LOOP ( 'NONE', ( #13002, #4729, #12451, #13194, #14956 ) ) ;
#20418=EDGE_LOOP ( 'NONE', ( #10944, #16278, #8416, #14353, #19585, #9603 ) ) ;
#20446=CARTESIAN_POINT ( 'NONE',  ( 1.713198289069999936, -17.44292009260000142, -147.5552959529999839 ) ) ;
#20447=EDGE_CURVE ( 'NONE', #19447, #21873, #13609, .T. ) ;
#20448=CARTESIAN_POINT ( 'NONE',  ( 5.631397321050000571, -17.85059010000000157, -147.5552959529999839 ) ) ;
#20454=CARTESIAN_POINT ( 'NONE',  ( 17.58326321919999558, -18.99156222550000095, -147.5552959529999839 ) ) ;
#20457=CARTESIAN_POINT ( 'NONE',  ( -10.01911575600000148, -21.69748113039999637, -147.5552959529999839 ) ) ;
#20460=CARTESIAN_POINT ( 'NONE',  ( 22.36721601470000209, -21.34320095609999868, -148.5552959529999839 ) ) ;
#20472=DIRECTION ( 'NONE',  ( 1.526468026911764926E-13, 8.159623473496129815E-13, 1.000000000000000000 ) ) ;
#20481=LINE ( 'NONE', #20600, #13871 ) ;
#20489=CARTESIAN_POINT ( 'NONE',  ( 1.561837858109999866, -18.84848306830000197, -143.5552959529999839 ) ) ;
#20495=CARTESIAN_POINT ( 'NONE',  ( -5.070907855429999778, -22.41528233759999722, -147.5552959529999839 ) ) ;
#20496=CARTESIAN_POINT ( 'NONE',  ( 16.26251912989999937, -22.62374141290000296, -144.5552959529999839 ) ) ;
#20497=LINE ( 'NONE', #4197, #20305 ) ;
#20499=ORIENTED_EDGE ( 'NONE', *, *, #13915, .F. ) ;
#20509=CARTESIAN_POINT ( 'NONE',  ( 5.276897646260000130, -21.39828525539999760, -144.5552959529999839 ) ) ;
#20514=LINE ( 'NONE', #4329, #2112 ) ;
#20519=VECTOR ( 'NONE', #11786, 1000.000000000000000 ) ;
#20522=CIRCLE ( 'NONE', #8345, 15.00000000000000000 ) ;
#20523=ORIENTED_EDGE ( 'NONE', *, *, #21074, .F. ) ;
#20535=VECTOR ( 'NONE', #18555, 1000.000000000000000 ) ;
#20536=VECTOR ( 'NONE', #18745, 999.9999999999998863 ) ;
#20541=ORIENTED_EDGE ( 'NONE', *, *, #10532, .F. ) ;
#20544=ORIENTED_EDGE ( 'NONE', *, *, #10004, .F. ) ;
#20545=ORIENTED_EDGE ( 'NONE', *, *, #17238, .F. ) ;
#20546=CARTESIAN_POINT ( 'NONE',  ( 22.36721601470000209, -21.34320095609999868, -148.0552959529999839 ) ) ;
#20549=VERTEX_POINT ( 'NONE', #13451 ) ;
#20555=CARTESIAN_POINT ( 'NONE',  ( 24.38136133040000075, -29.22855050349999928, -145.5552959529999839 ) ) ;
#20564=AXIS2_PLACEMENT_3D ( 'NONE', #16153, #19846, #1185 ) ;
#20576=DIRECTION ( 'NONE',  ( -8.955190032050000935E-12, 9.104778821549999739E-13, -1.000000000000000000 ) ) ;
#20592=EDGE_CURVE ( 'NONE', #20668, #15779, #5274, .T. ) ;
#20600=CARTESIAN_POINT ( 'NONE',  ( 25.00000852249999994, -26.83294714660000224, -143.0552959529999839 ) ) ;
#20605=VECTOR ( 'NONE', #12959, 999.9999999999998863 ) ;
#20609=VECTOR ( 'NONE', #22369, 1000.000000000000000 ) ;
#20611=CARTESIAN_POINT ( 'NONE',  ( -9.434278515689999978, -18.41834002140000237, -147.5552959529999839 ) ) ;
#20620=DIRECTION ( 'NONE',  ( 1.526468026912475027E-13, 8.159623473505000399E-13, 1.000000000000000000 ) ) ;
#20626=( NAMED_UNIT ( * ) PLANE_ANGLE_UNIT ( ) SI_UNIT ( $, .RADIAN. ) );
#20628=DIRECTION ( 'NONE',  ( -1.527666881879999979E-13, -8.171241461240000022E-13, -1.000000000000000000 ) ) ;
#20634=CARTESIAN_POINT ( 'NONE',  ( -6.657076963140000636, -20.13603737529999904, -145.5552959529999839 ) ) ;
#20637=EDGE_LOOP ( 'NONE', ( #16647, #9784, #3304, #23149, #20675, #16033 ) ) ;
#20638=STYLED_ITEM ( 'NONE', ( #13958 ), #1875 ) ;
#20640=EDGE_CURVE ( 'NONE', #14365, #4754, #17266, .T. ) ;
#20641=EDGE_CURVE ( 'NONE', #18669, #2618, #10230, .T. ) ;
#20649=ORIENTED_EDGE ( 'NONE', *, *, #13104, .T. ) ;
#20658=FACE_OUTER_BOUND ( 'NONE', #8939, .T. ) ;
#20668=VERTEX_POINT ( 'NONE', #21317 ) ;
#20675=ORIENTED_EDGE ( 'NONE', *, *, #10283, .F. ) ;
#20676=DIRECTION ( 'NONE',  ( -0.09606172499277226828, -0.9953753789357124848, 8.289665250527615055E-13 ) ) ;
#20679=VERTEX_POINT ( 'NONE', #9989 ) ;
#20680=AXIS2_PLACEMENT_3D ( 'NONE', #164, #18364, #3370 ) ;
#20684=CARTESIAN_POINT ( 'NONE',  ( 16.25412235410000150, -22.59491385829999999, -146.5552959529999839 ) ) ;
#20685=DIRECTION ( 'NONE',  ( 1.526468026909999897E-13, 8.159623473500000156E-13, 1.000000000000000000 ) ) ;
#20689=ORIENTED_EDGE ( 'NONE', *, *, #6586, .T. ) ;
#20690=LINE ( 'NONE', #18330, #7903 ) ;
#20693=ORIENTED_EDGE ( 'NONE', *, *, #8203, .F. ) ;
#20698=DIRECTION ( 'NONE',  ( 8.955190032050000935E-12, -9.104778821549999739E-13, 1.000000000000000000 ) ) ;
#20699=CARTESIAN_POINT ( 'NONE',  ( 8.915010983423528046, -17.39036197557994612, -144.5552959530300257 ) ) ;
#20700=VERTEX_POINT ( 'NONE', #1095 ) ;
#20711=CARTESIAN_POINT ( 'NONE',  ( 14.25179003943139655, -18.18074738980093130, -145.5552959530190833 ) ) ;
#20712=CARTESIAN_POINT ( 'NONE',  ( 20.40453940470000305, -31.75469340779999428, -144.5552959529999839 ) ) ;
#20714=FACE_OUTER_BOUND ( 'NONE', #3852, .T. ) ;
#20720=VECTOR ( 'NONE', #16061, 1000.000000000000227 ) ;
#20731=LINE ( 'NONE', #16715, #17789 ) ;
#20732=ORIENTED_EDGE ( 'NONE', *, *, #22197, .F. ) ;
#20741=EDGE_CURVE ( 'NONE', #18313, #19961, #1862, .T. ) ;
#20744=CYLINDRICAL_SURFACE ( 'NONE', #19268, 8.176568160359998672 ) ;
#20746=LINE ( 'NONE', #4212, #11269 ) ;
#20747=CARTESIAN_POINT ( 'NONE',  ( -8.296392858609999976, -9.821782169089999570, -147.5552959529999839 ) ) ;
#20780=ORIENTED_EDGE ( 'NONE', *, *, #16266, .F. ) ;
#20784=ORIENTED_EDGE ( 'NONE', *, *, #18623, .F. ) ;
#20785=CARTESIAN_POINT ( 'NONE',  ( -4.521812268179999705, -27.38504028299999860, -147.5552959529999839 ) ) ;
#20798=ORIENTED_EDGE ( 'NONE', *, *, #9407, .F. ) ;
#20799=VECTOR ( 'NONE', #10062, 1000.000000000000227 ) ;
#20805=FACE_OUTER_BOUND ( 'NONE', #8931, .T. ) ;
#20808=DIRECTION ( 'NONE',  ( 0.000000000000000000, 6.264364525598899972E-11, -1.000000000000000000 ) ) ;
#20813=EDGE_CURVE ( 'NONE', #18344, #12998, #7177, .T. ) ;
#20815=ORIENTED_EDGE ( 'NONE', *, *, #1490, .T. ) ;
#20816=FACE_OUTER_BOUND ( 'NONE', #6217, .T. ) ;
#20817=DIRECTION ( 'NONE',  ( 8.955190032049010580E-12, -9.104778821567928717E-13, 1.000000000000000000 ) ) ;
#20818=EDGE_LOOP ( 'NONE', ( #10040, #13131, #9416, #18367 ) ) ;
#20820=VERTEX_POINT ( 'NONE', #16308 ) ;
#20831=DIRECTION ( 'NONE',  ( 1.526468026909999897E-13, 8.159623473500000156E-13, 1.000000000000000000 ) ) ;
#20835=AXIS2_PLACEMENT_3D ( 'NONE', #14294, #21565, #21688 ) ;
#20837=DIRECTION ( 'NONE',  ( -0.1778629393740580045, -0.9840552701943220404, 3.562475540061165072E-13 ) ) ;
#20839=VECTOR ( 'NONE', #7905, 999.9999999999998863 ) ;
#20845=CARTESIAN_POINT ( 'NONE',  ( 24.38136133040000075, -29.22855050349999928, -146.5552959529999839 ) ) ;
#20851=CARTESIAN_POINT ( 'NONE',  ( 23.50000000000000000, -20.50000000000000000, -144.7152959530000089 ) ) ;
#20854=VECTOR ( 'NONE', #7467, 1000.000000000000000 ) ;
#20857=ADVANCED_FACE ( 'NONE', ( #7020 ), #21905, .T. ) ;
#20858=DIRECTION ( 'NONE',  ( 0.000000000000000000, -1.000000000000000000, 8.159623473500000156E-13 ) ) ;
#20863=AXIS2_PLACEMENT_3D ( 'NONE', #22143, #494, #5829 ) ;
#20867=DIRECTION ( 'NONE',  ( -0.9892101392001054760, 0.1465035852930155480, 4.471739159800472250E-12 ) ) ;
#20870=ORIENTED_EDGE ( 'NONE', *, *, #98, .F. ) ;
#20873=VECTOR ( 'NONE', #8355, 1000.000000000000000 ) ;
#20874=VERTEX_POINT ( 'NONE', #17978 ) ;
#20883=CARTESIAN_POINT ( 'NONE',  ( -6.635402838459999231, -21.69968975860000171, -146.5552959529999839 ) ) ;
#20885=ORIENTED_EDGE ( 'NONE', *, *, #9511, .T. ) ;
#20888=ADVANCED_FACE ( 'NONE', ( #16766 ), #14983, .T. ) ;
#20894=VECTOR ( 'NONE', #1681, 1000.000000000000227 ) ;
#20905=EDGE_LOOP ( 'NONE', ( #2363, #20026, #7635, #22720 ) ) ;
#20910=ORIENTED_EDGE ( 'NONE', *, *, #18884, .F. ) ;
#20913=ADVANCED_FACE ( 'NONE', ( #9610 ), #4041, .F. ) ;
#20915=LINE ( 'NONE', #15676, #18189 ) ;
#20922=PLANE ( 'NONE',  #8297 ) ;
#20928=ORIENTED_EDGE ( 'NONE', *, *, #1401, .T. ) ;
#20935=VERTEX_POINT ( 'NONE', #13189 ) ;
#20938=VERTEX_POINT ( 'NONE', #11165 ) ;
#20944=CARTESIAN_POINT ( 'NONE',  ( -8.916553640509999212, -11.88594259849999979, -143.5552959529999839 ) ) ;
#20955=CARTESIAN_POINT ( 'NONE',  ( 1.584389485034097822, -18.56644239314076117, -143.5552959530000692 ) ) ;
#20957=FACE_OUTER_BOUND ( 'NONE', #22558, .T. ) ;
#20971=EDGE_CURVE ( 'NONE', #7451, #11927, #4157, .T. ) ;
#20975=EDGE_CURVE ( 'NONE', #1657, #4706, #593, .T. ) ;
#20976=LINE ( 'NONE', #20845, #5863 ) ;
#20977=ORIENTED_EDGE ( 'NONE', *, *, #18827, .T. ) ;
#20980=CARTESIAN_POINT ( 'NONE',  ( -6.635402838469999232, -21.69968975860000171, -147.0552959529999839 ) ) ;
#20990=CARTESIAN_POINT ( 'NONE',  ( 9.152949117189999484, -16.59780702190000312, -148.0552959529999839 ) ) ;
#20992=CARTESIAN_POINT ( 'NONE',  ( 1.364575185789999923, -21.31553777220000256, -143.5552959529999839 ) ) ;
#20993=CARTESIAN_POINT ( 'NONE',  ( -7.149448239889999890, -25.45628515800000002, -145.5552959529999839 ) ) ;
#20995=ORIENTED_EDGE ( 'NONE', *, *, #20371, .T. ) ;
#21006=EDGE_CURVE ( 'NONE', #10871, #3534, #20690, .T. ) ;
#21010=LINE ( 'NONE', #11347, #9316 ) ;
#21047=LINE ( 'NONE', #20684, #18158 ) ;
#21065=DIRECTION ( 'NONE',  ( -0.1000233216789610108, -0.9949850929136109245, 3.559993607998610461E-13 ) ) ;
#21066=VERTEX_POINT ( 'NONE', #1309 ) ;
#21070=EDGE_LOOP ( 'NONE', ( #8256, #17416, #15932, #16302, #8629 ) ) ;
#21074=EDGE_CURVE ( 'NONE', #9406, #14014, #20115, .T. ) ;
#21079=DIRECTION ( 'NONE',  ( -0.9913873220698726785, 0.1309625047069831461, 0.000000000000000000 ) ) ;
#21083=DIRECTION ( 'NONE',  ( 2.842170943040000002E-14, 3.552713678800000097E-13, 1.000000000000000000 ) ) ;
#21086=LINE ( 'NONE', #23217, #10972 ) ;
#21087=CARTESIAN_POINT ( 'NONE',  ( -9.394779979509999990, -17.86685386420000299, -143.5552959529999839 ) ) ;
#21103=DIRECTION ( 'NONE',  ( -0.1000233216789610108, -0.9949850929136110356, 3.564252608777523239E-13 ) ) ;
#21105=AXIS2_PLACEMENT_3D ( 'NONE', #6772, #2982, #19157 ) ;
#21112=FILL_AREA_STYLE ('',( #2904 ) ) ;
#21116=CARTESIAN_POINT ( 'NONE',  ( -6.320468577110000652, -16.70961797440000041, -147.0552959529999839 ) ) ;
#21132=CYLINDRICAL_SURFACE ( 'NONE', #19586, 14.99999999999999467 ) ;
#21133=ORIENTED_EDGE ( 'NONE', *, *, #2533, .T. ) ;
#21143=VERTEX_POINT ( 'NONE', #13272 ) ;
#21146=ORIENTED_EDGE ( 'NONE', *, *, #8404, .F. ) ;
#21153=ADVANCED_FACE ( 'NONE', ( #323 ), #4120, .T. ) ;
#21160=LINE ( 'NONE', #17104, #17069 ) ;
#21163=CARTESIAN_POINT ( 'NONE',  ( -1.844824604570000082, -14.10750774809999974, -148.5552959529999839 ) ) ;
#21173=AXIS2_PLACEMENT_3D ( 'NONE', #18144, #11099, #5635 ) ;
#21183=LINE ( 'NONE', #10439, #343 ) ;
#21186=EDGE_CURVE ( 'NONE', #15988, #2866, #4593, .T. ) ;
#21188=EDGE_CURVE ( 'NONE', #6545, #11025, #6035, .T. ) ;
#21194=CARTESIAN_POINT ( 'NONE',  ( 25.04148309045456955, -26.71426189482850333, -147.5552959530288035 ) ) ;
#21204=CARTESIAN_POINT ( 'NONE',  ( -9.434278515689999978, -18.41834002140000237, -147.5552959529999839 ) ) ;
#21219=CARTESIAN_POINT ( 'NONE',  ( 2.218297500549999857, -15.44723318490000175, -147.5552959529999839 ) ) ;
#21221=DIRECTION ( 'NONE',  ( -0.07970438983373200059, -0.9968185442904001770, 8.268372250843320857E-13 ) ) ;
#21245=PLANE ( 'NONE',  #3815 ) ;
#21251=VECTOR ( 'NONE', #888, 1000.000000000000114 ) ;
#21254=AXIS2_PLACEMENT_3D ( 'NONE', #842, #20698, #18684 ) ;
#21256=VECTOR ( 'NONE', #5192, 1000.000000000000000 ) ;
#21262=EDGE_CURVE ( 'NONE', #11453, #19376, #17439, .T. ) ;
#21280=DIRECTION ( 'NONE',  ( -4.430318231639999944E-12, 6.100259101500000139E-13, -1.000000000000000000 ) ) ;
#21281=CARTESIAN_POINT ( 'NONE',  ( 25.02856554857857674, -26.78821141716894871, -146.5552959529967154 ) ) ;
#21286=ORIENTED_EDGE ( 'NONE', *, *, #18480, .T. ) ;
#21290=VECTOR ( 'NONE', #23209, 1000.000000000000114 ) ;
#21292=VERTEX_POINT ( 'NONE', #8263 ) ;
#21297=ORIENTED_EDGE ( 'NONE', *, *, #16367, .F. ) ;
#21299=DIRECTION ( 'NONE',  ( 4.430318231639999944E-12, -6.100259101500000139E-13, 1.000000000000000000 ) ) ;
#21305=( GEOMETRIC_REPRESENTATION_CONTEXT ( 3 ) GLOBAL_UNCERTAINTY_ASSIGNED_CONTEXT ( ( #18271 ) ) GLOBAL_UNIT_ASSIGNED_CONTEXT ( ( #18596, #20626, #14676 ) ) REPRESENTATION_CONTEXT ( 'NONE', 'WORKASPACE' ) );
#21311=DIRECTION ( 'NONE',  ( -2.842170943040000002E-14, -3.552713678800000097E-13, -1.000000000000000000 ) ) ;
#21317=CARTESIAN_POINT ( 'NONE',  ( 25.00000852249999994, -26.83294714660000224, -142.5552959529999839 ) ) ;
#21319=ORIENTED_EDGE ( 'NONE', *, *, #10682, .T. ) ;
#21322=LINE ( 'NONE', #13931, #6037 ) ;
#21326=DIRECTION ( 'NONE',  ( 0.2024296638729825848, 0.9792968044389154247, -3.528679552389696828E-13 ) ) ;
#21344=CIRCLE ( 'NONE', #22868, 5.000000000000000000 ) ;
#21349=DIRECTION ( 'NONE',  ( -2.043390161445605165E-12, 0.000000000000000000, -1.000000000000000000 ) ) ;
#21351=EDGE_CURVE ( 'NONE', #9207, #17699, #12271, .T. ) ;
#21354=ORIENTED_EDGE ( 'NONE', *, *, #7117, .T. ) ;
#21357=CARTESIAN_POINT ( 'NONE',  ( 24.87050155979999744, -26.86223000240000047, -146.5552959529999839 ) ) ;
#21369=LINE ( 'NONE', #1499, #10455 ) ;
#21370=DIRECTION ( 'NONE',  ( 1.527666881879999979E-13, 8.171241461240000022E-13, 1.000000000000000000 ) ) ;
#21372=DIRECTION ( 'NONE',  ( 4.510774274160000731E-12, -1.321907670990000086E-13, 1.000000000000000000 ) ) ;
#21375=ORIENTED_EDGE ( 'NONE', *, *, #23203, .F. ) ;
#21382=EDGE_LOOP ( 'NONE', ( #14929, #15800, #20367, #13855, #14490, #15778 ) ) ;
#21384=DIRECTION ( 'NONE',  ( 1.000000000000000000, 0.000000000000000000, -1.527536832333224173E-13 ) ) ;
#21403=DIRECTION ( 'NONE',  ( -7.483957154334591044E-15, 0.000000000000000000, 1.000000000000000000 ) ) ;
#21409=CARTESIAN_POINT ( 'NONE',  ( 20.40453940470000305, -31.75469340779999428, -143.5552959529999839 ) ) ;
#21410=EDGE_LOOP ( 'NONE', ( #14471, #10465, #8108, #14011 ) ) ;
#21416=DIRECTION ( 'NONE',  ( -0.06298685227120542907, -0.9980143568310855251, 1.534772309240130738E-13 ) ) ;
#21427=ORIENTED_EDGE ( 'NONE', *, *, #17136, .T. ) ;
#21428=DIRECTION ( 'NONE',  ( 4.433786671139999973E-12, -6.110667527539999876E-13, 1.000000000000000000 ) ) ;
#21442=DIRECTION ( 'NONE',  ( 1.000000000000000000, 0.000000000000000000, -8.954760363766765626E-12 ) ) ;
#21444=AXIS2_PLACEMENT_3D ( 'NONE', #12644, #19915, #10609 ) ;
#21449=CARTESIAN_POINT ( 'NONE',  ( 8.982728679470000088, -17.28848751049999777, -144.5552959529999839 ) ) ;
#21450=EDGE_LOOP ( 'NONE', ( #21146, #7738, #8851, #874, #14998, #15816, #15909, #1304 ) ) ;
#21458=PLANE ( 'NONE',  #9313 ) ;
#21467=FACE_OUTER_BOUND ( 'NONE', #12776, .T. ) ;
#21473=ORIENTED_EDGE ( 'NONE', *, *, #10111, .T. ) ;
#21475=EDGE_CURVE ( 'NONE', #21766, #12998, #18953, .T. ) ;
#21477=EDGE_CURVE ( 'NONE', #1038, #11485, #10128, .T. ) ;
#21480=LINE ( 'NONE', #21598, #9848 ) ;
#21483=EDGE_CURVE ( 'NONE', #22206, #16939, #10367, .T. ) ;
#21484=CARTESIAN_POINT ( 'NONE',  ( 9.152949117189999484, -16.59780702190000312, -147.5552959529999839 ) ) ;
#21487=FACE_OUTER_BOUND ( 'NONE', #3443, .T. ) ;
#21497=VERTEX_POINT ( 'NONE', #2666 ) ;
#21503=PLANE ( 'NONE',  #428 ) ;
#21505=CARTESIAN_POINT ( 'NONE',  ( -7.041959465309999722, -26.08051538799999847, -142.5552959529999839 ) ) ;
#21508=EDGE_CURVE ( 'NONE', #6588, #17682, #15502, .T. ) ;
#21513=ORIENTED_EDGE ( 'NONE', *, *, #6162, .F. ) ;
#21514=DIRECTION ( 'NONE',  ( 0.07970438983373200059, 0.9968185442904001770, -8.277822871613320832E-13 ) ) ;
#21533=PLANE ( 'NONE',  #13284 ) ;
#21539=ORIENTED_EDGE ( 'NONE', *, *, #3157, .F. ) ;
#21541=DIRECTION ( 'NONE',  ( 0.2229045288590935092, 0.9748402797454081004, -3.928002761761645078E-13 ) ) ;
#21554=B_SPLINE_CURVE_WITH_KNOTS ( 'NONE', 3,
 ( #6928, #15737, #12159, #10717 ),
 .UNSPECIFIED., .F., .F.,
 ( 4, 4 ),
 ( 0.000000000000000000, 1.000000000000000000 ),
 .UNSPECIFIED. ) ;
#21563=CARTESIAN_POINT ( 'NONE',  ( -4.192924954330000453, -28.60725908990000121, -146.5552959529999839 ) ) ;
#21565=DIRECTION ( 'NONE',  ( 8.955190032050000935E-12, -9.104778821549999739E-13, 1.000000000000000000 ) ) ;
#21569=DIRECTION ( 'NONE',  ( 4.430318231639999944E-12, -6.100259101500000139E-13, 1.000000000000000000 ) ) ;
#21575=ORIENTED_EDGE ( 'NONE', *, *, #19734, .T. ) ;
#21581=ORIENTED_EDGE ( 'NONE', *, *, #3145, .T. ) ;
#21587=CARTESIAN_POINT ( 'NONE',  ( -9.434278515689999978, -18.41834002140000237, -146.5552959529999839 ) ) ;
#21595=CIRCLE ( 'NONE', #20072, 14.99999999999999822 ) ;
#21598=CARTESIAN_POINT ( 'NONE',  ( 23.19105773460000108, -15.44374190390000123, -146.0552959529999839 ) ) ;
#21601=PLANE ( 'NONE',  #4834 ) ;
#21604=DIRECTION ( 'NONE',  ( 2.839308199620000013E-14, 3.568879590630000244E-13, 1.000000000000000000 ) ) ;
#21611=ADVANCED_FACE ( 'NONE', ( #11419 ), #3835, .T. ) ;
#21613=VERTEX_POINT ( 'NONE', #9629 ) ;
#21622=CARTESIAN_POINT ( 'NONE',  ( -6.320468577110000652, -16.70961797440000041, -146.5552959529999839 ) ) ;
#21627=VERTEX_POINT ( 'NONE', #263 ) ;
#21632=ORIENTED_EDGE ( 'NONE', *, *, #21186, .F. ) ;
#21633=VECTOR ( 'NONE', #22367, 999.9999999999998863 ) ;
#21636=ORIENTED_EDGE ( 'NONE', *, *, #7490, .T. ) ;
#21642=ORIENTED_EDGE ( 'NONE', *, *, #16367, .T. ) ;
#21646=CIRCLE ( 'NONE', #353, 8.176568160360000448 ) ;
#21659=LINE ( 'NONE', #1674, #3011 ) ;
#21661=LINE ( 'NONE', #14272, #13166 ) ;
#21662=VECTOR ( 'NONE', #14485, 1000.000000000000000 ) ;
#21663=CARTESIAN_POINT ( 'NONE',  ( 15.59498359470000040, -26.23371093219999750, -148.0552959529999839 ) ) ;
#21675=LINE ( 'NONE', #10452, #9170 ) ;
#21676=EDGE_CURVE ( 'NONE', #18387, #19018, #2635, .T. ) ;
#21680=VERTEX_POINT ( 'NONE', #15246 ) ;
#21688=DIRECTION ( 'NONE',  ( 1.000000000000000000, 0.000000000000000000, -8.955190032050000935E-12 ) ) ;
#21693=ORIENTED_EDGE ( 'NONE', *, *, #11781, .F. ) ;
#21704=EDGE_CURVE ( 'NONE', #13141, #8311, #15710, .T. ) ;
#21714=DIRECTION ( 'NONE',  ( -0.2208456705930775810, -0.9753087663813413410, 1.089717887850382194E-12 ) ) ;
#21720=VECTOR ( 'NONE', #12095, 1000.000000000000114 ) ;
#21724=LINE ( 'NONE', #6953, #4070 ) ;
#21733=VERTEX_POINT ( 'NONE', #8196 ) ;
#21736=DIRECTION ( 'NONE',  ( 1.526468026909999897E-13, 8.159623473500000156E-13, 1.000000000000000000 ) ) ;
#21738=CIRCLE ( 'NONE', #14882, 8.176568160360000448 ) ;
#21741=ADVANCED_FACE ( 'NONE', ( #15468 ), #22972, .F. ) ;
#21747=ORIENTED_EDGE ( 'NONE', *, *, #15416, .T. ) ;
#21749=ADVANCED_FACE ( 'NONE', ( #9866 ), #12010, .T. ) ;
#21754=VECTOR ( 'NONE', #20405, 999.9999999999998863 ) ;
#21755=ADVANCED_FACE ( 'NONE', ( #6657 ), #17140, .T. ) ;
#21757=CARTESIAN_POINT ( 'NONE',  ( 16.62554907222028078, -18.90013506635313334, -146.5552959530255350 ) ) ;
#21759=CARTESIAN_POINT ( 'NONE',  ( -7.129475577410000042, -25.57825421080000083, -143.5552959529999839 ) ) ;
#21766=VERTEX_POINT ( 'NONE', #13444 ) ;
#21774=LINE ( 'NONE', #12282, #10250 ) ;
#21775=EDGE_CURVE ( 'NONE', #11995, #13663, #18807, .T. ) ;
#21776=VECTOR ( 'NONE', #19509, 1000.000000000000114 ) ;
#21786=LINE ( 'NONE', #14390, #20720 ) ;
#21802=EDGE_LOOP ( 'NONE', ( #4520, #2267, #7772, #19309 ) ) ;
#21803=DIRECTION ( 'NONE',  ( -8.955058916629999092E-12, 9.112710586119999183E-13, -1.000000000000000000 ) ) ;
#21808=EDGE_CURVE ( 'NONE', #20679, #10162, #15177, .T. ) ;
#21816=ORIENTED_EDGE ( 'NONE', *, *, #13915, .T. ) ;
#21824=DIRECTION ( 'NONE',  ( 2.839308199620000013E-14, 3.568879590630000244E-13, 1.000000000000000000 ) ) ;
#21825=CARTESIAN_POINT ( 'NONE',  ( 24.85988213910000155, -26.16224997189999968, -145.5552959529999839 ) ) ;
#21827=ORIENTED_EDGE ( 'NONE', *, *, #20971, .F. ) ;
#21830=ORIENTED_EDGE ( 'NONE', *, *, #4003, .T. ) ;
#21832=CARTESIAN_POINT ( 'NONE',  ( 23.21181482502162297, -23.48612613680712968, -142.5552959529975112 ) ) ;
#21864=EDGE_CURVE ( 'NONE', #8311, #15451, #15943, .T. ) ;
#21873=VERTEX_POINT ( 'NONE', #21194 ) ;
#21874=CARTESIAN_POINT ( 'NONE',  ( -6.320468577110000652, -16.70961797440000041, -147.5552959529999839 ) ) ;
#21877=CARTESIAN_POINT ( 'NONE',  ( 6.959824834146532524, -28.67531053199257229, -145.5552959530214991 ) ) ;
#21878=ORIENTED_EDGE ( 'NONE', *, *, #20315, .T. ) ;
#21885=DIRECTION ( 'NONE',  ( 1.000000000000000000, 0.000000000000000000, -4.430318231639999944E-12 ) ) ;
#21886=PLANE ( 'NONE',  #22759 ) ;
#21889=AXIS2_PLACEMENT_3D ( 'NONE', #67, #22070, #5636 ) ;
#21890=EDGE_CURVE ( 'NONE', #1427, #7689, #17725, .T. ) ;
#21892=DIRECTION ( 'NONE',  ( -0.1435602414469281940, -0.9896415801065048257, 3.847089866708073804E-13 ) ) ;
#21894=CARTESIAN_POINT ( 'NONE',  ( -9.282104535860000283, -16.71402168319999859, -145.5552959529999839 ) ) ;
#21905=PLANE ( 'NONE',  #22368 ) ;
#21906=AXIS2_PLACEMENT_3D ( 'NONE', #14010, #23176, #21403 ) ;
#21907=VECTOR ( 'NONE', #22502, 1000.000000000000000 ) ;
#21923=ORIENTED_EDGE ( 'NONE', *, *, #9526, .T. ) ;
#21927=VERTEX_POINT ( 'NONE', #12953 ) ;
#21935=ADVANCED_FACE ( 'NONE', ( #16876 ), #14866, .T. ) ;
#21937=PLANE ( 'NONE',  #5405 ) ;
#21939=CARTESIAN_POINT ( 'NONE',  ( -9.347107914279998653, -17.32706600430000066, -144.5552959529999839 ) ) ;
#21942=ORIENTED_EDGE ( 'NONE', *, *, #2416, .F. ) ;
#21944=FILL_AREA_STYLE_COLOUR ( '', #17488 ) ;
#21952=CARTESIAN_POINT ( 'NONE',  ( -9.334216945200001447, -17.19633444960000190, -145.5552959529999839 ) ) ;
#21964=CARTESIAN_POINT ( 'NONE',  ( 23.17093239529999948, -15.44501179329999907, -144.5552959529999839 ) ) ;
#21983=VERTEX_POINT ( 'NONE', #20454 ) ;
#21984=DIRECTION ( 'NONE',  ( 4.510774274160000731E-12, -1.321907670990000086E-13, 1.000000000000000000 ) ) ;
#21986=ORIENTED_EDGE ( 'NONE', *, *, #6924, .T. ) ;
#21992=CARTESIAN_POINT ( 'NONE',  ( 1.172620240290000115, -63.19354141059999108, -146.5552959529999839 ) ) ;
#21993=AXIS2_PLACEMENT_3D ( 'NONE', #9161, #5246, #3826 ) ;
#21994=AXIS2_PLACEMENT_3D ( 'NONE', #13282, #4255, #7807 ) ;
#22012=DIRECTION ( 'NONE',  ( 1.526468026909860048E-13, 8.159623473498529972E-13, 1.000000000000000000 ) ) ;
#22015=CARTESIAN_POINT ( 'NONE',  ( 16.65421564080000039, -18.61497348660000029, -146.0552959529999839 ) ) ;
#22016=VECTOR ( 'NONE', #4711, 1000.000000000000114 ) ;
#22019=AXIS2_PLACEMENT_3D ( 'NONE', #15832, #10110, #17385 ) ;
#22021=DIRECTION ( 'NONE',  ( 0.4289374931909490374, 0.9033341723498921061, -8.025326435147559991E-13 ) ) ;
#22022=DIRECTION ( 'NONE',  ( 1.000000000000000000, 0.000000000000000000, -8.955190032050000935E-12 ) ) ;
#22025=DIRECTION ( 'NONE',  ( 4.510170015240000199E-12, -1.314504061159999897E-13, 1.000000000000000000 ) ) ;
#22026=ADVANCED_FACE ( 'NONE', ( #6517 ), #13413, .T. ) ;
#22029=VECTOR ( 'NONE', #17163, 1000.000000000000000 ) ;
#22030=VECTOR ( 'NONE', #8317, 1000.000000000000114 ) ;
#22031=ORIENTED_EDGE ( 'NONE', *, *, #9777, .F. ) ;
#22037=AXIS2_PLACEMENT_3D ( 'NONE', #22255, #20472, #4169 ) ;
#22043=LINE ( 'NONE', #9985, #15789 ) ;
#22046=CARTESIAN_POINT ( 'NONE',  ( 16.82730212879999598, -31.88969284570000084, -146.5552959529999839 ) ) ;
#22052=CARTESIAN_POINT ( 'NONE',  ( -8.679997173036046121, -12.46618270809291396, -147.5552959529663610 ) ) ;
#22056=AXIS2_PLACEMENT_3D ( 'NONE', #9068, #11319, #14916 ) ;
#22070=DIRECTION ( 'NONE',  ( -0.9968185442904002880, 0.07970438983373201447, 8.712538262633493651E-14 ) ) ;
#22073=EDGE_LOOP ( 'NONE', ( #20541, #10405, #16537, #5044 ) ) ;
#22079=DIRECTION ( 'NONE',  ( -4.511946372079999833E-12, 1.314504061159999897E-13, -1.000000000000000000 ) ) ;
#22092=ORIENTED_EDGE ( 'NONE', *, *, #10539, .T. ) ;
#22098=VERTEX_POINT ( 'NONE', #8051 ) ;
#22105=ORIENTED_EDGE ( 'NONE', *, *, #2416, .T. ) ;
#22112=CARTESIAN_POINT ( 'NONE',  ( 24.59017985859999911, -26.91621017459999976, -148.0552959529999839 ) ) ;
#22115=AXIS2_PLACEMENT_3D ( 'NONE', #22801, #18989, #19219 ) ;
#22117=VECTOR ( 'NONE', #747, 1000.000000000000114 ) ;
#22119=CARTESIAN_POINT ( 'NONE',  ( 5.792747474889999637, -16.92794981449999980, -144.5552959529999839 ) ) ;
#22135=ORIENTED_EDGE ( 'NONE', *, *, #18029, .F. ) ;
#22139=CARTESIAN_POINT ( 'NONE',  ( 15.85402906740000084, -26.57485422999999969, -146.0552959529999839 ) ) ;
#22143=CARTESIAN_POINT ( 'NONE',  ( 2.531727043920000142, -11.80034048859999807, -148.5552959529999839 ) ) ;
#22146=COLOUR_RGB ( '', 0.66274510, 0.83137255, 0.94901961) ;
#22147=EDGE_CURVE ( 'NONE', #20820, #6134, #2601, .T. ) ;
#22149=VECTOR ( 'NONE', #2315, 1000.000000000000227 ) ;
#22185=ADVANCED_FACE ( 'NONE', ( #1535 ), #4971, .F. ) ;
#22197=EDGE_CURVE ( 'NONE', #21733, #15113, #9894, .T. ) ;
#22206=VERTEX_POINT ( 'NONE', #6743 ) ;
#22208=ORIENTED_EDGE ( 'NONE', *, *, #14598, .F. ) ;
#22213=AXIS2_PLACEMENT_3D ( 'NONE', #18099, #11058, #1810 ) ;
#22227=ORIENTED_EDGE ( 'NONE', *, *, #7732, .T. ) ;
#22230=DIRECTION ( 'NONE',  ( -1.526468026909999897E-13, -8.159623473500000156E-13, -1.000000000000000000 ) ) ;
#22238=CARTESIAN_POINT ( 'NONE',  ( 24.55924402540000173, -29.20875385929999979, -143.5552959529999839 ) ) ;
#22243=DIRECTION ( 'NONE',  ( -7.483957154334591044E-15, 0.000000000000000000, 1.000000000000000000 ) ) ;
#22248=LINE ( 'NONE', #20120, #5350 ) ;
#22255=CARTESIAN_POINT ( 'NONE',  ( 22.40884248670000289, -21.39641658300000060, -144.0552959529999839 ) ) ;
#22256=ORIENTED_EDGE ( 'NONE', *, *, #2994, .F. ) ;
#22257=DIRECTION ( 'NONE',  ( 0.000000000000000000, -1.000000000000000000, 8.159623473500000156E-13 ) ) ;
#22261=DIRECTION ( 'NONE',  ( 2.839308199620000013E-14, 3.568879590630000244E-13, 1.000000000000000000 ) ) ;
#22269=DIRECTION ( 'NONE',  ( -0.07970438983373200059, -0.9968185442904001770, 8.268372250843320857E-13 ) ) ;
#22273=ADVANCED_FACE ( 'NONE', ( #8415 ), #5324, .F. ) ;
#22276=DIRECTION ( 'NONE',  ( 4.510774274160000731E-12, -1.321907670990000086E-13, 1.000000000000000000 ) ) ;
#22277=EDGE_CURVE ( 'NONE', #18690, #4598, #22465, .T. ) ;
#22283=VECTOR ( 'NONE', #1378, 1000.000000000000000 ) ;
#22287=LINE ( 'NONE', #20509, #13259 ) ;
#22294=EDGE_CURVE ( 'NONE', #12155, #7923, #8632, .T. ) ;
#22296=ORIENTED_EDGE ( 'NONE', *, *, #948, .F. ) ;
#22315=EDGE_LOOP ( 'NONE', ( #17244, #11508, #2350, #17420 ) ) ;
#22318=CARTESIAN_POINT ( 'NONE',  ( 15.85402906740000084, -26.57485422999999969, -146.5552959529999839 ) ) ;
#22322=VECTOR ( 'NONE', #732, 1000.000000000000000 ) ;
#22329=VERTEX_POINT ( 'NONE', #21757 ) ;
#22331=ORIENTED_EDGE ( 'NONE', *, *, #959, .F. ) ;
#22342=VECTOR ( 'NONE', #7289, 1000.000000000000000 ) ;
#22344=AXIS2_PLACEMENT_3D ( 'NONE', #6251, #4467, #13752 ) ;
#22350=CARTESIAN_POINT ( 'NONE',  ( -8.296392858609999976, -9.821782169089999570, -148.0552959529999839 ) ) ;
#22365=FACE_OUTER_BOUND ( 'NONE', #11501, .T. ) ;
#22367=DIRECTION ( 'NONE',  ( -0.09606172499277226828, -0.9953753789357124848, 8.289665250527615055E-13 ) ) ;
#22368=AXIS2_PLACEMENT_3D ( 'NONE', #12483, #10807, #23329 ) ;
#22369=DIRECTION ( 'NONE',  ( -0.1435602414469281940, -0.9896415801065048257, 3.847089866708073804E-13 ) ) ;
#22373=DIRECTION ( 'NONE',  ( 1.000000000000000000, 0.000000000000000000, -1.522591576628786004E-13 ) ) ;
#22402=SURFACE_SIDE_STYLE ('',( #7411 ) ) ;
#22407=LINE ( 'NONE', #13357, #23162 ) ;
#22417=ORIENTED_EDGE ( 'NONE', *, *, #13867, .F. ) ;
#22418=AXIS2_PLACEMENT_3D ( 'NONE', #4933, #17418, #13966 ) ;
#22421=CIRCLE ( 'NONE', #7544, 15.00000000000000000 ) ;
#22422=VERTEX_POINT ( 'NONE', #9332 ) ;
#22425=LINE ( 'NONE', #13137, #8511 ) ;
#22429=ORIENTED_EDGE ( 'NONE', *, *, #3909, .F. ) ;
#22432=VECTOR ( 'NONE', #3690, 999.9999999999998863 ) ;
#22447=ORIENTED_EDGE ( 'NONE', *, *, #10655, .F. ) ;
#22455=CARTESIAN_POINT ( 'NONE',  ( -6.049191701419999845, -14.51144913589999952, -146.0552959529999839 ) ) ;
#22459=ORIENTED_EDGE ( 'NONE', *, *, #16522, .T. ) ;
#22465=CIRCLE ( 'NONE', #10295, 5.000000000000000000 ) ;
#22472=EDGE_LOOP ( 'NONE', ( #13680, #21827, #16604, #7319, #5564 ) ) ;
#22477=ORIENTED_EDGE ( 'NONE', *, *, #4032, .F. ) ;
#22478=CARTESIAN_POINT ( 'NONE',  ( -8.734077015120000453, -11.22642389220000148, -146.5552959529999839 ) ) ;
#22485=LINE ( 'NONE', #23279, #5718 ) ;
#22488=LINE ( 'NONE', #18559, #20609 ) ;
#22491=AXIS2_PLACEMENT_3D ( 'NONE', #20153, #20268, #16804 ) ;
#22494=ADVANCED_FACE ( 'NONE', ( #7902 ), #13954, .T. ) ;
#22495=CARTESIAN_POINT ( 'NONE',  ( -9.394779979509999990, -17.86685386420000299, -142.5552959529999839 ) ) ;
#22500=EDGE_LOOP ( 'NONE', ( #9983, #23088, #8162, #2958 ) ) ;
#22502=DIRECTION ( 'NONE',  ( -1.525446435830000185E-13, -8.171241461240000022E-13, -1.000000000000000000 ) ) ;
#22504=DIRECTION ( 'NONE',  ( -0.1000233216789610108, -0.9949850929136109245, 3.576398436658600095E-13 ) ) ;
#22505=VERTEX_POINT ( 'NONE', #22318 ) ;
#22507=VECTOR ( 'NONE', #2125, 1000.000000000000114 ) ;
#22508=DIRECTION ( 'NONE',  ( -0.9913873220698726785, 0.1309625047069831461, -1.853446743629759619E-14 ) ) ;
#22511=DIRECTION ( 'NONE',  ( -0.9892101392001054760, 0.1465035852930155480, 4.471739159800472250E-12 ) ) ;
#22518=ORIENTED_EDGE ( 'NONE', *, *, #5801, .F. ) ;
#22533=ADVANCED_FACE ( 'NONE', ( #4238 ), #13266, .T. ) ;
#22537=VERTEX_POINT ( 'NONE', #6694 ) ;
#22538=CARTESIAN_POINT ( 'NONE',  ( -8.665242998822469289, -11.36832253183628616, -144.5552959529994439 ) ) ;
#22541=FACE_OUTER_BOUND ( 'NONE', #22315, .T. ) ;
#22547=LINE ( 'NONE', #6825, #7220 ) ;
#22549=EDGE_CURVE ( 'NONE', #19018, #13428, #13499, .T. ) ;
#22550=VERTEX_POINT ( 'NONE', #19313 ) ;
#22553=VERTEX_POINT ( 'NONE', #18867 ) ;
#22558=EDGE_LOOP ( 'NONE', ( #13022, #4294, #4124, #22092, #7048 ) ) ;
#22561=EDGE_LOOP ( 'NONE', ( #22331, #2185, #4625, #3818, #1902, #17587, #18996, #5507, #1987, #21286, #2078 ) ) ;
#22562=PLANE ( 'NONE',  #19306 ) ;
#22573=LINE ( 'NONE', #11369, #7579 ) ;
#22581=PLANE ( 'NONE',  #9826 ) ;
#22582=LINE ( 'NONE', #8161, #5309 ) ;
#22583=ORIENTED_EDGE ( 'NONE', *, *, #21808, .T. ) ;
#22584=VECTOR ( 'NONE', #22629, 1000.000000000000000 ) ;
#22587=ORIENTED_EDGE ( 'NONE', *, *, #14577, .F. ) ;
#22602=EDGE_CURVE ( 'NONE', #8980, #17699, #17531, .T. ) ;
#22603=DIRECTION ( 'NONE',  ( -1.527666881879999979E-13, -8.153477892850000134E-13, -1.000000000000000000 ) ) ;
#22607=VERTEX_POINT ( 'NONE', #13388 ) ;
#22608=EDGE_CURVE ( 'NONE', #21873, #6936, #2352, .T. ) ;
#22616=DIRECTION ( 'NONE',  ( 0.04856869991388110264, 0.9988198443106121038, -3.578457907868606044E-13 ) ) ;
#22618=LINE ( 'NONE', #6202, #13981 ) ;
#22628=DIRECTION ( 'NONE',  ( 8.955190032050000935E-12, -9.104778821549999739E-13, 1.000000000000000000 ) ) ;
#22629=DIRECTION ( 'NONE',  ( -0.1435602414469281940, -0.9896415801065048257, 3.849849731938073961E-13 ) ) ;
#22631=CARTESIAN_POINT ( 'NONE',  ( 23.93619342817335394, -31.59589658247995203, -143.5552959530006660 ) ) ;
#22634=ORIENTED_EDGE ( 'NONE', *, *, #792, .F. ) ;
#22658=DIRECTION ( 'NONE',  ( 4.430318231639999944E-12, -6.100259101500000139E-13, 1.000000000000000000 ) ) ;
#22675=DIRECTION ( 'NONE',  ( 0.3704939739869947957, -0.9288348697369861462, -4.163336342344337834E-12 ) ) ;
#22698=ORIENTED_EDGE ( 'NONE', *, *, #377, .F. ) ;
#22705=ORIENTED_EDGE ( 'NONE', *, *, #16572, .F. ) ;
#22713=ORIENTED_EDGE ( 'NONE', *, *, #3995, .F. ) ;
#22714=DIRECTION ( 'NONE',  ( 4.510774274160000731E-12, -1.321907670990000086E-13, 1.000000000000000000 ) ) ;
#22720=ORIENTED_EDGE ( 'NONE', *, *, #17299, .F. ) ;
#22725=DIRECTION ( 'NONE',  ( -0.9846904924346531196, 0.1743118874569385135, 0.000000000000000000 ) ) ;
#22734=CARTESIAN_POINT ( 'NONE',  ( 23.89222110089999873, -31.59487100459999809, -146.0552959529999839 ) ) ;
#22736=VERTEX_POINT ( 'NONE', #22046 ) ;
#22739=ADVANCED_FACE ( 'NONE', ( #622 ), #11536, .T. ) ;
#22744=PLANE ( 'NONE',  #12645 ) ;
#22753=FACE_OUTER_BOUND ( 'NONE', #21410, .T. ) ;
#22759=AXIS2_PLACEMENT_3D ( 'NONE', #20094, #17838, #1556 ) ;
#22773=CARTESIAN_POINT ( 'NONE',  ( 23.17093239529999948, -15.44501179329999907, -143.5552959529999839 ) ) ;
#22774=ADVANCED_FACE ( 'NONE', ( #3840 ), #2302, .T. ) ;
#22777=VECTOR ( 'NONE', #21892, 1000.000000000000000 ) ;
#22796=CIRCLE ( 'NONE', #17859, 35.00000000000000000 ) ;
#22798=CARTESIAN_POINT ( 'NONE',  ( 16.61718498210000305, -18.75502267109999721, -142.5552959529999839 ) ) ;
#22801=CARTESIAN_POINT ( 'NONE',  ( 1.172620240290000115, -63.19354141059999108, -145.5552959529999839 ) ) ;
#22805=CARTESIAN_POINT ( 'NONE',  ( -6.405315633307901990, -18.05400298756394406, -146.5552959530004387 ) ) ;
#22813=CIRCLE ( 'NONE', #4180, 6.000000000000001776 ) ;
#22814=CARTESIAN_POINT ( 'NONE',  ( 16.33424841169999908, -31.58611763329999889, -148.0552959529999839 ) ) ;
#22817=CARTESIAN_POINT ( 'NONE',  ( 24.36715301250000110, -30.57462384669999977, -146.5552959529999839 ) ) ;
#22821=FACE_OUTER_BOUND ( 'NONE', #16228, .T. ) ;
#22822=CARTESIAN_POINT ( 'NONE',  ( -9.334216945200001447, -17.19633444960000190, -146.5552959529999839 ) ) ;
#22823=VERTEX_POINT ( 'NONE', #13693 ) ;
#22831=CARTESIAN_POINT ( 'NONE',  ( -8.770737564319999180, -11.35481373070000011, -144.0552959529999839 ) ) ;
#22839=ORIENTED_EDGE ( 'NONE', *, *, #22608, .T. ) ;
#22840=LINE ( 'NONE', #4986, #18984 ) ;
#22841=CARTESIAN_POINT ( 'NONE',  ( -8.734077015120000453, -11.22642389220000148, -146.5552959529999839 ) ) ;
#22846=ADVANCED_FACE ( 'NONE', ( #11772 ), #17378, .T. ) ;
#22847=CARTESIAN_POINT ( 'NONE',  ( 22.42591623494620023, -15.34961090601114542, -144.5552959529997281 ) ) ;
#22849=EDGE_CURVE ( 'NONE', #12998, #6817, #19048, .T. ) ;
#22850=ORIENTED_EDGE ( 'NONE', *, *, #23402, .T. ) ;
#22851=AXIS2_PLACEMENT_3D ( 'NONE', #17648, #11475, #18753 ) ;
#22861=EDGE_CURVE ( 'NONE', #5977, #16716, #9988, .T. ) ;
#22868=AXIS2_PLACEMENT_3D ( 'NONE', #16372, #21736, #19938 ) ;
#22873=LINE ( 'NONE', #15725, #11175 ) ;
#22876=LINE ( 'NONE', #17392, #19880 ) ;
#22880=ORIENTED_EDGE ( 'NONE', *, *, #20741, .T. ) ;
#22885=DIRECTION ( 'NONE',  ( -0.9840552701943220404, 0.1778629393740580045, 0.000000000000000000 ) ) ;
#22887=AXIS2_PLACEMENT_3D ( 'NONE', #19534, #22984, #15606 ) ;
#22904=DIRECTION ( 'NONE',  ( 0.2024296638729825848, 0.9792968044389154247, -3.528679552389696828E-13 ) ) ;
#22907=ORIENTED_EDGE ( 'NONE', *, *, #6208, .F. ) ;
#22910=CARTESIAN_POINT ( 'NONE',  ( 4.128836048070000153, -25.17057797350000214, -148.5552959529999839 ) ) ;
#22913=EDGE_CURVE ( 'NONE', #16792, #21766, #10228, .T. ) ;
#22943=CARTESIAN_POINT ( 'NONE',  ( -4.888913597060000171, -24.24628707910000003, -143.0552959529999839 ) ) ;
#22945=DIRECTION ( 'NONE',  ( 2.839308199620000013E-14, 3.568879590630000244E-13, 1.000000000000000000 ) ) ;
#22947=DIRECTION ( 'NONE',  ( 2.839308199620000013E-14, 3.568879590630000244E-13, 1.000000000000000000 ) ) ;
#22953=PLANE ( 'NONE',  #3499 ) ;
#22964=LINE ( 'NONE', #17605, #13289 ) ;
#22970=DIRECTION ( 'NONE',  ( 4.500711553433139826E-12, 0.000000000000000000, 1.000000000000000000 ) ) ;
#22972=PLANE ( 'NONE',  #23164 ) ;
#22976=FACE_OUTER_BOUND ( 'NONE', #12338, .T. ) ;
#22983=PLANE ( 'NONE',  #22019 ) ;
#22984=DIRECTION ( 'NONE',  ( -0.1465035852930155202, -0.9892101392001055871, 4.561368942930487546E-14 ) ) ;
#22988=FACE_OUTER_BOUND ( 'NONE', #4864, .T. ) ;
#23006=VECTOR ( 'NONE', #19833, 1000.000000000000114 ) ;
#23007=ORIENTED_EDGE ( 'NONE', *, *, #9511, .F. ) ;
#23009=SURFACE_STYLE_USAGE ( .BOTH. , #17411 ) ;
#23015=ORIENTED_EDGE ( 'NONE', *, *, #10655, .T. ) ;
#23016=DIRECTION ( 'NONE',  ( 1.000000000000000000, 0.000000000000000000, -1.526556658859589738E-13 ) ) ;
#23020=VERTEX_POINT ( 'NONE', #14047 ) ;
#23028=FACE_OUTER_BOUND ( 'NONE', #13223, .T. ) ;
#23040=ORIENTED_EDGE ( 'NONE', *, *, #18531, .F. ) ;
#23043=EDGE_CURVE ( 'NONE', #22550, #19256, #21675, .T. ) ;
#23051=AXIS2_PLACEMENT_3D ( 'NONE', #15115, #22261, #13329 ) ;
#23055=DIRECTION ( 'NONE',  ( 0.000000000000000000, -1.000000000000000000, 3.568879590630000244E-13 ) ) ;
#23056=ORIENTED_EDGE ( 'NONE', *, *, #17057, .T. ) ;
#23058=EDGE_CURVE ( 'NONE', #7250, #10198, #17856, .T. ) ;
#23070=ORIENTED_EDGE ( 'NONE', *, *, #1412, .T. ) ;
#23074=DIRECTION ( 'NONE',  ( 1.000000000000000000, 0.000000000000000000, -1.526556658859589738E-13 ) ) ;
#23076=DIRECTION ( 'NONE',  ( 1.000000000000000000, 0.000000000000000000, -4.430318231639999944E-12 ) ) ;
#23077=EDGE_CURVE ( 'NONE', #4115, #21983, #8792, .T. ) ;
#23079=PLANE ( 'NONE',  #18554 ) ;
#23080=AXIS2_PLACEMENT_3D ( 'NONE', #8843, #3975, #15029 ) ;
#23085=PLANE ( 'NONE',  #21105 ) ;
#23088=ORIENTED_EDGE ( 'NONE', *, *, #9952, .T. ) ;
#23099=DIRECTION ( 'NONE',  ( -0.07970438983373200059, -0.9968185442904001770, 8.265980492683321082E-13 ) ) ;
#23100=PLANE ( 'NONE',  #11088 ) ;
#23101=LINE ( 'NONE', #6791, #552 ) ;
#23103=DIRECTION ( 'NONE',  ( 0.6183952767652367566, -0.7858672163123019416, -2.891205793294677010E-12 ) ) ;
#23109=DIRECTION ( 'NONE',  ( -0.9847555042252370550, 0.1739442350240419932, 1.062521554950256121E-14 ) ) ;
#23113=DIRECTION ( 'NONE',  ( -4.510774274160000731E-12, 1.321907670990000086E-13, -1.000000000000000000 ) ) ;
#23114=AXIS2_PLACEMENT_3D ( 'NONE', #21759, #6866, #14135 ) ;
#23117=VERTEX_POINT ( 'NONE', #13187 ) ;
#23122=ORIENTED_EDGE ( 'NONE', *, *, #21351, .T. ) ;
#23123=LINE ( 'NONE', #3144, #9529 ) ;
#23134=VECTOR ( 'NONE', #5819, 1000.000000000000114 ) ;
#23137=EDGE_CURVE ( 'NONE', #12827, #18274, #9264, .T. ) ;
#23144=CARTESIAN_POINT ( 'NONE',  ( 17.58326321919999558, -18.99156222550000095, -147.0552959529999839 ) ) ;
#23145=CARTESIAN_POINT ( 'NONE',  ( -9.923478264230000789, -23.29931827799999766, -144.0552959529999839 ) ) ;
#23149=ORIENTED_EDGE ( 'NONE', *, *, #17578, .F. ) ;
#23159=CARTESIAN_POINT ( 'NONE',  ( -9.282104535860000283, -16.71402168319999859, -145.5552959529999839 ) ) ;
#23162=VECTOR ( 'NONE', #20628, 1000.000000000000000 ) ;
#23164=AXIS2_PLACEMENT_3D ( 'NONE', #6197, #17016, #22725 ) ;
#23166=EDGE_CURVE ( 'NONE', #10162, #13656, #16429, .T. ) ;
#23173=CARTESIAN_POINT ( 'NONE',  ( -9.334216945200001447, -17.19633444960000190, -146.5552959529999839 ) ) ;
#23176=DIRECTION ( 'NONE',  ( -0.9949850929136110356, 0.1000233216789610247, -7.446425804567087094E-15 ) ) ;
#23188=EDGE_CURVE ( 'NONE', #17671, #16792, #14981, .T. ) ;
#23199=ORIENTED_EDGE ( 'NONE', *, *, #1503, .T. ) ;
#23203=EDGE_CURVE ( 'NONE', #16847, #21680, #13371, .T. ) ;
#23209=DIRECTION ( 'NONE',  ( -0.9892101392001054760, 0.1465035852930155480, 4.471739159800472250E-12 ) ) ;
#23215=EDGE_CURVE ( 'NONE', #20361, #11545, #16882, .T. ) ;
#23217=CARTESIAN_POINT ( 'NONE',  ( 24.75935218339999722, -28.32938697159999819, -146.5552959529999839 ) ) ;
#23218=EDGE_CURVE ( 'NONE', #3418, #14604, #18675, .T. ) ;
#23220=CARTESIAN_POINT ( 'NONE',  ( -9.334216945200001447, -17.19633444960000190, -145.5552959529999839 ) ) ;
#23227=LINE ( 'NONE', #20980, #6010 ) ;
#23233=DIRECTION ( 'NONE',  ( 4.510774274160000731E-12, -1.321907670990000086E-13, 1.000000000000000000 ) ) ;
#23237=CIRCLE ( 'NONE', #9911, 15.00000000000000178 ) ;
#23239=AXIS2_PLACEMENT_3D ( 'NONE', #1283, #10404, #21384 ) ;
#23240=DIRECTION ( 'NONE',  ( 0.2451800884060535979, 0.9694775522152123681, -1.317373699560290683E-12 ) ) ;
#23244=( LENGTH_UNIT ( ) NAMED_UNIT ( * ) SI_UNIT ( .MILLI., .METRE. ) );
#23248=CARTESIAN_POINT ( 'NONE',  ( 22.42370904790000097, -21.41421288319999761, -143.5552959529999839 ) ) ;
#23251=FACE_OUTER_BOUND ( 'NONE', #16474, .T. ) ;
#23254=AXIS2_PLACEMENT_3D ( 'NONE', #17414, #11685, #1137 ) ;
#23258=DIRECTION ( 'NONE',  ( 1.000000000000000000, 0.000000000000000000, -1.527536832333223921E-13 ) ) ;
#23269=VECTOR ( 'NONE', #8098, 1000.000000000000114 ) ;
#23273=ADVANCED_FACE ( 'NONE', ( #16994 ), #22953, .F. ) ;
#23278=CARTESIAN_POINT ( 'NONE',  ( 1.357896944629999991, -19.89221232270000073, -147.5552959529999839 ) ) ;
#23279=CARTESIAN_POINT ( 'NONE',  ( 24.89581725840000104, -26.85672394480000236, -144.0552959529999839 ) ) ;
#23286=DIRECTION ( 'NONE',  ( 2.839308199620000013E-14, 3.568879590630000244E-13, 1.000000000000000000 ) ) ;
#23308=CARTESIAN_POINT ( 'NONE',  ( -9.282104535849999394, -16.71402168319999859, -144.5552959529999839 ) ) ;
#23329=DIRECTION ( 'NONE',  ( 0.000000000000000000, -1.000000000000000000, 3.568879590630000244E-13 ) ) ;
#23330=EDGE_CURVE ( 'NONE', #1998, #17682, #1193, .T. ) ;
#23338=ORIENTED_EDGE ( 'NONE', *, *, #8983, .F. ) ;
#23341=EDGE_CURVE ( 'NONE', #20820, #4706, #8057, .T. ) ;
#23352=ORIENTED_EDGE ( 'NONE', *, *, #11263, .T. ) ;
#23361=FACE_OUTER_BOUND ( 'NONE', #17105, .T. ) ;
#23363=ORIENTED_EDGE ( 'NONE', *, *, #10626, .T. ) ;
#23364=DIRECTION ( 'NONE',  ( -4.537894428437109619E-14, 0.000000000000000000, 1.000000000000000000 ) ) ;
#23373=LINE ( 'NONE', #14678, #632 ) ;
#23376=LINE ( 'NONE', #23144, #11589 ) ;
#23381=CARTESIAN_POINT ( 'NONE',  ( 24.41610067590000099, -29.22497285029999858, -143.5552959529999839 ) ) ;
#23391=VECTOR ( 'NONE', #14680, 1000.000000000000000 ) ;
#23399=PLANE ( 'NONE',  #3829 ) ;
#23400=ORIENTED_EDGE ( 'NONE', *, *, #15785, .F. ) ;
#23402=EDGE_CURVE ( 'NONE', #21143, #6545, #6750, .T. ) ;
#23414=VERTEX_POINT ( 'NONE', #5330 ) ;
#23416=CARTESIAN_POINT ( 'NONE',  ( -9.350215169903842494, -17.08637274644199522, -147.5552959529998134 ) ) ;
#23439=CARTESIAN_POINT ( 'NONE',  ( -7.149448239889999890, -25.45628515800000002, -146.0552959529999839 ) ) ;
#23441=DIRECTION ( 'NONE',  ( 1.000000000000000000, 0.000000000000000000, -4.430318231639999944E-12 ) ) ;
#23443=CARTESIAN_POINT ( 'NONE',  ( 17.45728951470000112, -20.98759093920000041, -147.5552959529999839 ) ) ;
#23456=VERTEX_POINT ( 'NONE', #14013 ) ;
#23465=ORIENTED_EDGE ( 'NONE', *, *, #14838, .F. ) ;
#23468=AXIS2_PLACEMENT_3D ( 'NONE', #9981, #9865, #4648 ) ;
#23473=DIRECTION ( 'NONE',  ( 4.430318231636070029E-12, -6.100259101526210011E-13, 1.000000000000000000 ) ) ;
#23474=ORIENTED_EDGE ( 'NONE', *, *, #3682, .T. ) ;
#23476=DIRECTION ( 'NONE',  ( 1.000000000000000000, 0.000000000000000000, -4.430318231639999944E-12 ) ) ;
#23484=DIRECTION ( 'NONE',  ( 0.000000000000000000, 7.657380550038349542E-13, -1.000000000000000000 ) ) ;
#23486=EDGE_CURVE ( 'NONE', #5559, #1590, #3305, .T. ) ;
#23492=DIRECTION ( 'NONE',  ( -0.04169410462551791791, 0.9991304227374304681, -3.553937932771528679E-13 ) ) ;
#23495=CARTESIAN_POINT ( 'NONE',  ( 20.35976161480000002, -31.74228192520000391, -146.5552959529999839 ) ) ;
#23501=VERTEX_POINT ( 'NONE', #21874 ) ;
#23505=DIRECTION ( 'NONE',  ( -0.9938526945756316344, 0.1107105301439589573, 6.178155812097707047E-14 ) ) ;
#23513=CARTESIAN_POINT ( 'NONE',  ( 17.21087225569999646, -22.66053313549999970, -144.5552959529999839 ) ) ;
#23527=VECTOR ( 'NONE', #21065, 1000.000000000000227 ) ;
#23529=ORIENTED_EDGE ( 'NONE', *, *, #22147, .F. ) ;
#23537=ORIENTED_EDGE ( 'NONE', *, *, #9279, .T. ) ;
#23539=EDGE_CURVE ( 'NONE', #8887, #2628, #11459, .T. ) ;
ENDSEC;
END-ISO-10303-21;
